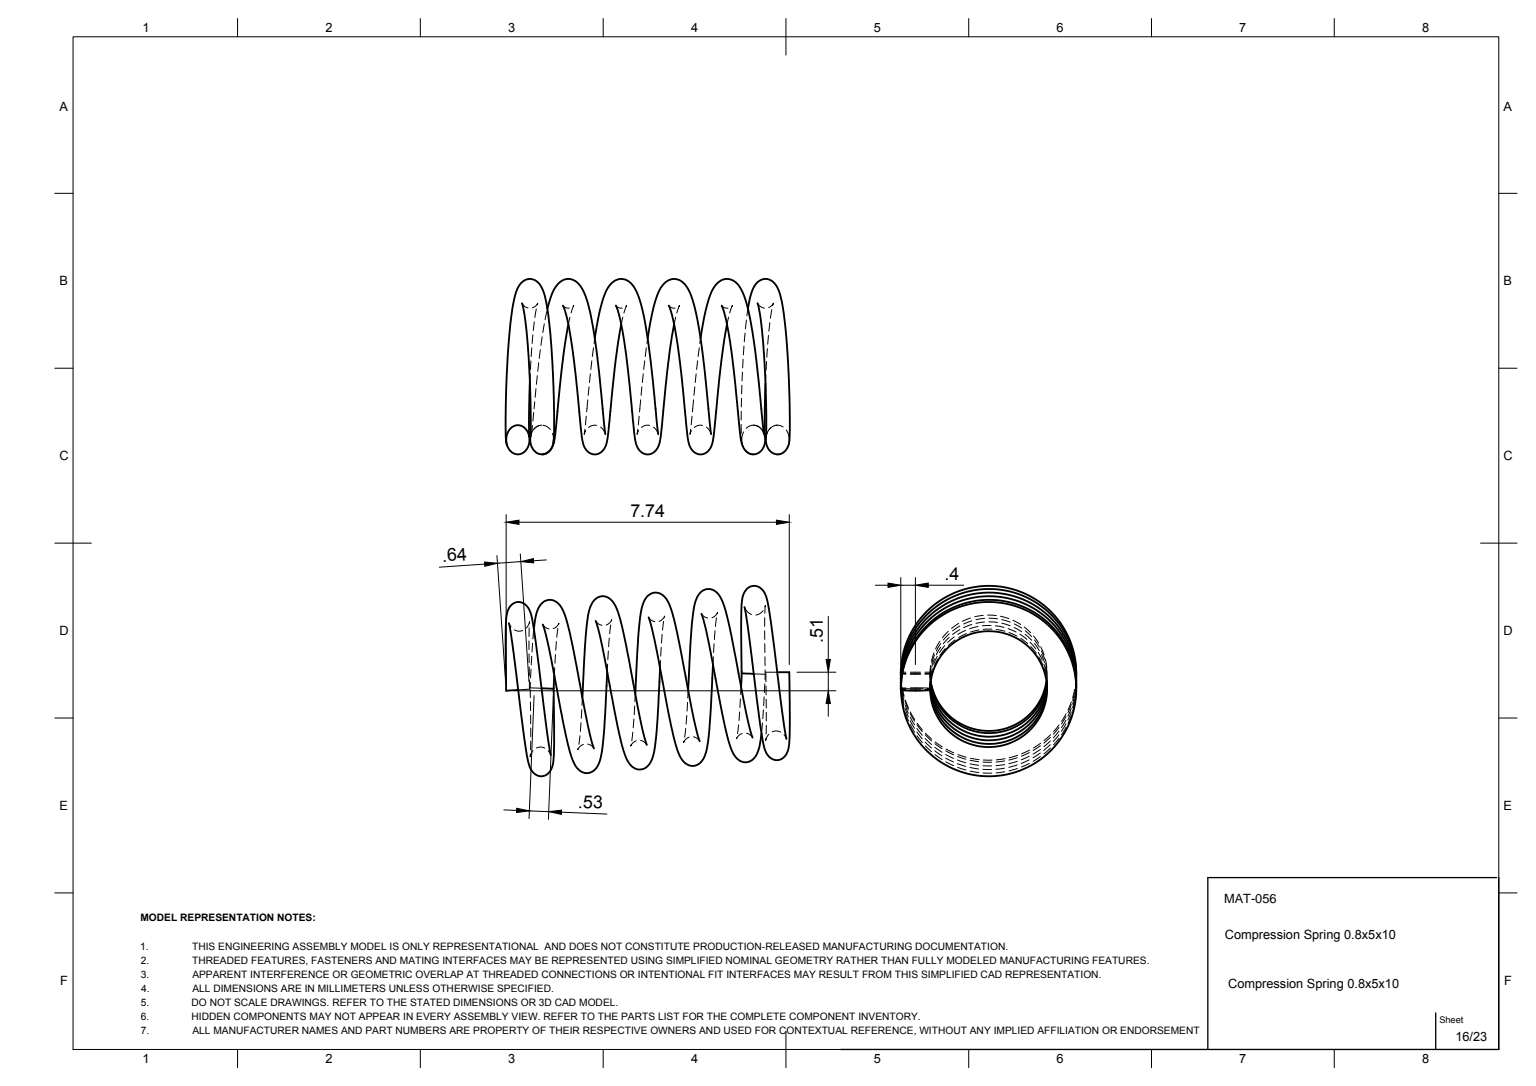
ISO-10303-21;
HEADER;
/* Generated by software containing ST-Developer
 * from STEP Tools, Inc. (www.steptools.com) 
 */

FILE_DESCRIPTION(
/* description */ (''),
/* implementation_level */ '2;1');

FILE_NAME(
/* name */ 'Compression Spring 0.8x5x10.step',
/* time_stamp */ '2026-10-28T16:47:13+01:00',
/* author */ (''),
/* organization */ (''),
/* preprocessor_version */ 'ST-DEVELOPER v20.2',
/* originating_system */ 'Autodesk Translation Framework v15.17.0.0',
/* authorisation */ '');

FILE_SCHEMA (('AUTOMOTIVE_DESIGN { 1 0 10303 214 3 1 1 }'));
ENDSEC;

DATA;
#10=MECHANICAL_DESIGN_GEOMETRIC_PRESENTATION_REPRESENTATION('',(#4588),#459242);
#186=ELLIPSE('',#99155,0.40000000018352,0.321902553589955);
#187=ELLIPSE('',#99156,0.400000000332434,0.321319291807333);
#188=ELLIPSE('',#99157,0.40000000018352,0.321902553589955);
#189=ELLIPSE('',#99158,0.400000000010015,0.321902553729585);
#190=ELLIPSE('',#99159,0.400000000010015,0.321902553729585);
#191=ELLIPSE('',#99160,0.4,0.32);
#192=ELLIPSE('',#99161,0.4,0.32);
#193=ELLIPSE('',#99162,0.400000000010016,0.321902553729585);
#194=ELLIPSE('',#99163,0.400000000010016,0.321902553729585);
#195=ELLIPSE('',#99165,0.400000000183514,0.321902553589955);
#196=ELLIPSE('',#99166,0.400000000183514,0.321902553589955);
#197=ELLIPSE('',#99168,0.40000000033243,0.321319291807334);
#2309=(
BOUNDED_SURFACE()
B_SPLINE_SURFACE(3,3,((#363644,#363645,#363646,#363647,#363648,#363649,
#363650,#363651,#363652,#363653,#363654,#363655,#363656,#363657,#363658,
#363659,#363660,#363661,#363662,#363663,#363664,#363665,#363666,#363667,
#363668,#363669,#363670,#363671,#363672),(#363673,#363674,#363675,#363676,
#363677,#363678,#363679,#363680,#363681,#363682,#363683,#363684,#363685,
#363686,#363687,#363688,#363689,#363690,#363691,#363692,#363693,#363694,
#363695,#363696,#363697,#363698,#363699,#363700,#363701),(#363702,#363703,
#363704,#363705,#363706,#363707,#363708,#363709,#363710,#363711,#363712,
#363713,#363714,#363715,#363716,#363717,#363718,#363719,#363720,#363721,
#363722,#363723,#363724,#363725,#363726,#363727,#363728,#363729,#363730),
(#363731,#363732,#363733,#363734,#363735,#363736,#363737,#363738,#363739,
#363740,#363741,#363742,#363743,#363744,#363745,#363746,#363747,#363748,
#363749,#363750,#363751,#363752,#363753,#363754,#363755,#363756,#363757,
#363758,#363759),(#363760,#363761,#363762,#363763,#363764,#363765,#363766,
#363767,#363768,#363769,#363770,#363771,#363772,#363773,#363774,#363775,
#363776,#363777,#363778,#363779,#363780,#363781,#363782,#363783,#363784,
#363785,#363786,#363787,#363788),(#363789,#363790,#363791,#363792,#363793,
#363794,#363795,#363796,#363797,#363798,#363799,#363800,#363801,#363802,
#363803,#363804,#363805,#363806,#363807,#363808,#363809,#363810,#363811,
#363812,#363813,#363814,#363815,#363816,#363817),(#363818,#363819,#363820,
#363821,#363822,#363823,#363824,#363825,#363826,#363827,#363828,#363829,
#363830,#363831,#363832,#363833,#363834,#363835,#363836,#363837,#363838,
#363839,#363840,#363841,#363842,#363843,#363844,#363845,#363846)),
 .UNSPECIFIED.,.T.,.F.,.F.)
B_SPLINE_SURFACE_WITH_KNOTS((4,3,4),(4,1,1,1,1,1,1,1,1,1,1,1,1,1,1,1,1,
1,1,1,1,1,1,1,1,1,4),(0.,0.5,1.),(0.,0.0310703336761616,0.0624385278003938,
0.0937144048499659,0.124978469089869,0.166663774179581,0.208294236860357,
0.249966520356582,0.291641529650434,0.3332733240007,0.374947073344913,0.416620808022619,
0.458253030541402,0.499926784452264,0.54160045129851,0.583232674441905,
0.624906496125386,0.666580158626562,0.708211959489969,0.749887054558503,
0.791559255246094,0.833189756589646,0.87487513422873,0.906139159779086,
0.937415106668169,0.968783217665703,1.),.UNSPECIFIED.)
GEOMETRIC_REPRESENTATION_ITEM()
RATIONAL_B_SPLINE_SURFACE(((1.,1.,1.,1.,1.,1.,1.,1.,1.,1.,1.,1.,1.,1.,1.,
1.,1.,1.,1.,1.,1.,1.,1.,1.,1.,1.,1.,1.,1.),(0.333333333333333,0.333333333333333,
0.333333333333334,0.333333333333333,0.333333333333333,0.333333333333333,
0.333333333333333,0.333333333333333,0.333333333333333,0.333333333333333,
0.333333333333333,0.333333333333333,0.333333333333334,0.333333333333333,
0.333333333333333,0.333333333333333,0.333333333333333,0.333333333333333,
0.333333333333333,0.333333333333333,0.333333333333333,0.333333333333333,
0.333333333333333,0.333333333333333,0.333333333333333,0.333333333333333,
0.333333333333333,0.333333333333333,0.333333333333333),(0.333333333333333,
0.333333333333333,0.333333333333334,0.333333333333333,0.333333333333333,
0.333333333333333,0.333333333333333,0.333333333333333,0.333333333333333,
0.333333333333333,0.333333333333333,0.333333333333333,0.333333333333334,
0.333333333333333,0.333333333333333,0.333333333333333,0.333333333333333,
0.333333333333333,0.333333333333333,0.333333333333333,0.333333333333333,
0.333333333333333,0.333333333333333,0.333333333333333,0.333333333333333,
0.333333333333333,0.333333333333333,0.333333333333333,0.333333333333333),
(1.,1.,1.,1.,1.,1.,1.,1.,1.,1.,1.,1.,1.,1.,1.,1.,1.,1.,1.,1.,1.,1.,1.,1.,
1.,1.,1.,1.,1.),(0.333333333333333,0.333333333333333,0.333333333333334,
0.333333333333333,0.333333333333333,0.333333333333333,0.333333333333333,
0.333333333333333,0.333333333333333,0.333333333333333,0.333333333333333,
0.333333333333333,0.333333333333334,0.333333333333333,0.333333333333333,
0.333333333333333,0.333333333333333,0.333333333333333,0.333333333333333,
0.333333333333333,0.333333333333333,0.333333333333333,0.333333333333333,
0.333333333333333,0.333333333333333,0.333333333333333,0.333333333333333,
0.333333333333333,0.333333333333333),(0.333333333333333,0.333333333333333,
0.333333333333334,0.333333333333333,0.333333333333333,0.333333333333333,
0.333333333333333,0.333333333333333,0.333333333333333,0.333333333333333,
0.333333333333333,0.333333333333333,0.333333333333334,0.333333333333333,
0.333333333333333,0.333333333333333,0.333333333333333,0.333333333333333,
0.333333333333333,0.333333333333333,0.333333333333333,0.333333333333333,
0.333333333333333,0.333333333333333,0.333333333333333,0.333333333333333,
0.333333333333333,0.333333333333333,0.333333333333333),(1.,1.,1.,1.,1.,
1.,1.,1.,1.,1.,1.,1.,1.,1.,1.,1.,1.,1.,1.,1.,1.,1.,1.,1.,1.,1.,1.,1.,1.)))
REPRESENTATION_ITEM('')
SURFACE()
);
#2310=(
BOUNDED_SURFACE()
B_SPLINE_SURFACE(3,3,((#363913,#363914,#363915,#363916,#363917,#363918,
#363919,#363920,#363921,#363922,#363923,#363924,#363925,#363926,#363927,
#363928,#363929,#363930,#363931,#363932,#363933,#363934,#363935,#363936,
#363937,#363938,#363939,#363940,#363941,#363942,#363943,#363944,#363945,
#363946,#363947,#363948,#363949,#363950,#363951,#363952,#363953,#363954,
#363955,#363956,#363957,#363958,#363959,#363960,#363961,#363962,#363963,
#363964,#363965,#363966,#363967,#363968,#363969,#363970,#363971,#363972,
#363973,#363974,#363975,#363976,#363977,#363978,#363979,#363980,#363981,
#363982,#363983,#363984,#363985,#363986,#363987,#363988,#363989,#363990,
#363991,#363992,#363993,#363994,#363995,#363996,#363997,#363998,#363999,
#364000,#364001,#364002,#364003,#364004,#364005,#364006,#364007,#364008,
#364009,#364010,#364011),(#364012,#364013,#364014,#364015,#364016,#364017,
#364018,#364019,#364020,#364021,#364022,#364023,#364024,#364025,#364026,
#364027,#364028,#364029,#364030,#364031,#364032,#364033,#364034,#364035,
#364036,#364037,#364038,#364039,#364040,#364041,#364042,#364043,#364044,
#364045,#364046,#364047,#364048,#364049,#364050,#364051,#364052,#364053,
#364054,#364055,#364056,#364057,#364058,#364059,#364060,#364061,#364062,
#364063,#364064,#364065,#364066,#364067,#364068,#364069,#364070,#364071,
#364072,#364073,#364074,#364075,#364076,#364077,#364078,#364079,#364080,
#364081,#364082,#364083,#364084,#364085,#364086,#364087,#364088,#364089,
#364090,#364091,#364092,#364093,#364094,#364095,#364096,#364097,#364098,
#364099,#364100,#364101,#364102,#364103,#364104,#364105,#364106,#364107,
#364108,#364109,#364110),(#364111,#364112,#364113,#364114,#364115,#364116,
#364117,#364118,#364119,#364120,#364121,#364122,#364123,#364124,#364125,
#364126,#364127,#364128,#364129,#364130,#364131,#364132,#364133,#364134,
#364135,#364136,#364137,#364138,#364139,#364140,#364141,#364142,#364143,
#364144,#364145,#364146,#364147,#364148,#364149,#364150,#364151,#364152,
#364153,#364154,#364155,#364156,#364157,#364158,#364159,#364160,#364161,
#364162,#364163,#364164,#364165,#364166,#364167,#364168,#364169,#364170,
#364171,#364172,#364173,#364174,#364175,#364176,#364177,#364178,#364179,
#364180,#364181,#364182,#364183,#364184,#364185,#364186,#364187,#364188,
#364189,#364190,#364191,#364192,#364193,#364194,#364195,#364196,#364197,
#364198,#364199,#364200,#364201,#364202,#364203,#364204,#364205,#364206,
#364207,#364208,#364209),(#364210,#364211,#364212,#364213,#364214,#364215,
#364216,#364217,#364218,#364219,#364220,#364221,#364222,#364223,#364224,
#364225,#364226,#364227,#364228,#364229,#364230,#364231,#364232,#364233,
#364234,#364235,#364236,#364237,#364238,#364239,#364240,#364241,#364242,
#364243,#364244,#364245,#364246,#364247,#364248,#364249,#364250,#364251,
#364252,#364253,#364254,#364255,#364256,#364257,#364258,#364259,#364260,
#364261,#364262,#364263,#364264,#364265,#364266,#364267,#364268,#364269,
#364270,#364271,#364272,#364273,#364274,#364275,#364276,#364277,#364278,
#364279,#364280,#364281,#364282,#364283,#364284,#364285,#364286,#364287,
#364288,#364289,#364290,#364291,#364292,#364293,#364294,#364295,#364296,
#364297,#364298,#364299,#364300,#364301,#364302,#364303,#364304,#364305,
#364306,#364307,#364308),(#364309,#364310,#364311,#364312,#364313,#364314,
#364315,#364316,#364317,#364318,#364319,#364320,#364321,#364322,#364323,
#364324,#364325,#364326,#364327,#364328,#364329,#364330,#364331,#364332,
#364333,#364334,#364335,#364336,#364337,#364338,#364339,#364340,#364341,
#364342,#364343,#364344,#364345,#364346,#364347,#364348,#364349,#364350,
#364351,#364352,#364353,#364354,#364355,#364356,#364357,#364358,#364359,
#364360,#364361,#364362,#364363,#364364,#364365,#364366,#364367,#364368,
#364369,#364370,#364371,#364372,#364373,#364374,#364375,#364376,#364377,
#364378,#364379,#364380,#364381,#364382,#364383,#364384,#364385,#364386,
#364387,#364388,#364389,#364390,#364391,#364392,#364393,#364394,#364395,
#364396,#364397,#364398,#364399,#364400,#364401,#364402,#364403,#364404,
#364405,#364406,#364407),(#364408,#364409,#364410,#364411,#364412,#364413,
#364414,#364415,#364416,#364417,#364418,#364419,#364420,#364421,#364422,
#364423,#364424,#364425,#364426,#364427,#364428,#364429,#364430,#364431,
#364432,#364433,#364434,#364435,#364436,#364437,#364438,#364439,#364440,
#364441,#364442,#364443,#364444,#364445,#364446,#364447,#364448,#364449,
#364450,#364451,#364452,#364453,#364454,#364455,#364456,#364457,#364458,
#364459,#364460,#364461,#364462,#364463,#364464,#364465,#364466,#364467,
#364468,#364469,#364470,#364471,#364472,#364473,#364474,#364475,#364476,
#364477,#364478,#364479,#364480,#364481,#364482,#364483,#364484,#364485,
#364486,#364487,#364488,#364489,#364490,#364491,#364492,#364493,#364494,
#364495,#364496,#364497,#364498,#364499,#364500,#364501,#364502,#364503,
#364504,#364505,#364506),(#364507,#364508,#364509,#364510,#364511,#364512,
#364513,#364514,#364515,#364516,#364517,#364518,#364519,#364520,#364521,
#364522,#364523,#364524,#364525,#364526,#364527,#364528,#364529,#364530,
#364531,#364532,#364533,#364534,#364535,#364536,#364537,#364538,#364539,
#364540,#364541,#364542,#364543,#364544,#364545,#364546,#364547,#364548,
#364549,#364550,#364551,#364552,#364553,#364554,#364555,#364556,#364557,
#364558,#364559,#364560,#364561,#364562,#364563,#364564,#364565,#364566,
#364567,#364568,#364569,#364570,#364571,#364572,#364573,#364574,#364575,
#364576,#364577,#364578,#364579,#364580,#364581,#364582,#364583,#364584,
#364585,#364586,#364587,#364588,#364589,#364590,#364591,#364592,#364593,
#364594,#364595,#364596,#364597,#364598,#364599,#364600,#364601,#364602,
#364603,#364604,#364605)),.UNSPECIFIED.,.T.,.F.,.F.)
B_SPLINE_SURFACE_WITH_KNOTS((4,3,4),(4,1,1,1,1,1,1,1,1,1,1,1,1,1,1,1,1,
1,1,1,1,1,1,1,1,1,1,1,1,1,1,1,1,1,1,1,1,1,1,1,1,1,1,1,1,1,1,1,1,1,1,1,1,
1,1,1,1,1,1,1,1,1,1,1,1,1,1,1,1,1,1,1,1,1,1,1,1,1,1,1,1,1,1,1,1,1,1,1,1,
1,1,1,1,1,1,1,4),(0.,0.5,1.),(0.,0.0104467457848562,0.0208697051534179,
0.0312830741812588,0.0417059245369557,0.0521151844214314,0.0625350854994869,
0.072955523619078,0.0833651614361216,0.093785355257659,0.104205506224069,
0.114615259182489,0.125035444608255,0.135455580151817,0.145865343296126,
0.156285526040368,0.166705661591602,0.177115425208493,0.187535607700786,
0.197955743339009,0.208365506953668,0.218785689432554,0.229205825080053,
0.239615588692213,0.250035771170918,0.260455906818944,0.270865670430874,
0.281285852909622,0.291705988557657,0.302115752169577,0.312535934648329,
0.322956070296362,0.333365833908282,0.343786016387035,0.354206152035067,
0.364615915646988,0.375036098125741,0.385456233773773,0.395865997385694,
0.406286179864446,0.416706315512479,0.427116079124399,0.437536261603152,
0.447956397251184,0.458366160863105,0.468786343341857,0.47920647898989,
0.48961624260181,0.500036425080563,0.510456560728595,0.520866324340516,
0.531286506819269,0.541706642467301,0.552116406079222,0.562536588557974,
0.572956724206007,0.583366487817927,0.59378667029668,0.604206805944712,
0.614616569556633,0.625036752035385,0.635456887683418,0.645866651295338,
0.656286833774091,0.666706969422123,0.677116733034044,0.687536915512797,
0.697957051160829,0.708366814772749,0.718786997251504,0.729207132899531,
0.739616896511461,0.750037078990207,0.760457214638192,0.770866978250353,
0.781287160728572,0.791707296376735,0.802117059991444,0.812537242460403,
0.822957378121908,0.833367141740239,0.843787324122365,0.85420746003523,
0.864617223206175,0.875037405580635,0.885457544175532,0.895867297492078,
0.906287495257385,0.916707642366043,0.927117283641006,0.937537767903979,
0.947957624414904,0.958366904818021,0.968789794286159,0.979203137018726,
0.989626134310512,1.),.UNSPECIFIED.)
GEOMETRIC_REPRESENTATION_ITEM()
RATIONAL_B_SPLINE_SURFACE(((1.,1.,1.,1.,1.,1.,1.,1.,1.,1.,1.,1.,1.,1.,1.,
1.,1.,1.,1.,1.,1.,1.,1.,1.,1.,1.,1.,1.,1.,1.,1.,1.,1.,1.,1.,1.,1.,1.,1.,
1.,1.,1.,1.,1.,1.,1.,1.,1.,1.,1.,1.,1.,1.,1.,1.,1.,1.,1.,1.,1.,1.,1.,1.,
1.,1.,1.,1.,1.,1.,1.,1.,1.,1.,1.,1.,1.,1.,1.,1.,1.,1.,1.,1.,1.,1.,1.,1.,
1.,1.,1.,1.,1.,1.,1.,1.,1.,1.,1.,1.),(0.333333333333333,0.333333333333333,
0.333333333333333,0.333333333333333,0.333333333333333,0.333333333333333,
0.333333333333333,0.333333333333333,0.333333333333333,0.333333333333333,
0.333333333333333,0.333333333333333,0.333333333333333,0.333333333333333,
0.333333333333333,0.333333333333333,0.333333333333333,0.333333333333333,
0.333333333333333,0.333333333333333,0.333333333333333,0.333333333333333,
0.333333333333333,0.333333333333333,0.333333333333333,0.333333333333333,
0.333333333333333,0.333333333333333,0.333333333333333,0.333333333333333,
0.333333333333333,0.333333333333333,0.333333333333333,0.333333333333333,
0.333333333333333,0.333333333333333,0.333333333333333,0.333333333333333,
0.333333333333333,0.333333333333333,0.333333333333333,0.333333333333333,
0.333333333333333,0.333333333333333,0.333333333333333,0.333333333333333,
0.333333333333333,0.333333333333333,0.333333333333333,0.333333333333333,
0.333333333333333,0.333333333333333,0.333333333333333,0.333333333333333,
0.333333333333333,0.333333333333333,0.333333333333333,0.333333333333333,
0.333333333333333,0.333333333333333,0.333333333333333,0.333333333333333,
0.333333333333333,0.333333333333333,0.333333333333333,0.333333333333333,
0.333333333333333,0.333333333333333,0.333333333333333,0.333333333333333,
0.333333333333333,0.333333333333333,0.333333333333333,0.333333333333333,
0.333333333333333,0.333333333333333,0.333333333333333,0.333333333333333,
0.333333333333333,0.333333333333333,0.333333333333333,0.333333333333333,
0.333333333333333,0.333333333333333,0.333333333333333,0.333333333333333,
0.333333333333333,0.333333333333333,0.333333333333333,0.333333333333333,
0.333333333333333,0.333333333333333,0.333333333333333,0.333333333333333,
0.333333333333333,0.333333333333333,0.333333333333333,0.333333333333333,
0.333333333333333),(0.333333333333333,0.333333333333333,0.333333333333333,
0.333333333333333,0.333333333333333,0.333333333333333,0.333333333333333,
0.333333333333333,0.333333333333333,0.333333333333333,0.333333333333333,
0.333333333333333,0.333333333333333,0.333333333333333,0.333333333333333,
0.333333333333333,0.333333333333333,0.333333333333333,0.333333333333333,
0.333333333333333,0.333333333333333,0.333333333333333,0.333333333333333,
0.333333333333333,0.333333333333333,0.333333333333333,0.333333333333333,
0.333333333333333,0.333333333333333,0.333333333333333,0.333333333333333,
0.333333333333333,0.333333333333333,0.333333333333333,0.333333333333333,
0.333333333333333,0.333333333333333,0.333333333333333,0.333333333333333,
0.333333333333333,0.333333333333333,0.333333333333333,0.333333333333333,
0.333333333333333,0.333333333333333,0.333333333333333,0.333333333333333,
0.333333333333333,0.333333333333333,0.333333333333333,0.333333333333333,
0.333333333333333,0.333333333333333,0.333333333333333,0.333333333333333,
0.333333333333333,0.333333333333333,0.333333333333333,0.333333333333333,
0.333333333333333,0.333333333333333,0.333333333333333,0.333333333333333,
0.333333333333333,0.333333333333333,0.333333333333333,0.333333333333333,
0.333333333333333,0.333333333333333,0.333333333333333,0.333333333333333,
0.333333333333333,0.333333333333333,0.333333333333333,0.333333333333333,
0.333333333333333,0.333333333333333,0.333333333333333,0.333333333333333,
0.333333333333333,0.333333333333333,0.333333333333333,0.333333333333333,
0.333333333333333,0.333333333333333,0.333333333333333,0.333333333333333,
0.333333333333333,0.333333333333333,0.333333333333333,0.333333333333333,
0.333333333333333,0.333333333333333,0.333333333333333,0.333333333333333,
0.333333333333333,0.333333333333333,0.333333333333333,0.333333333333333),
(1.,1.,1.,1.,1.,1.,1.,1.,1.,1.,1.,1.,1.,1.,1.,1.,1.,1.,1.,1.,1.,1.,1.,1.,
1.,1.,1.,1.,1.,1.,1.,1.,1.,1.,1.,1.,1.,1.,1.,1.,1.,1.,1.,1.,1.,1.,1.,1.,
1.,1.,1.,1.,1.,1.,1.,1.,1.,1.,1.,1.,1.,1.,1.,1.,1.,1.,1.,1.,1.,1.,1.,1.,
1.,1.,1.,1.,1.,1.,1.,1.,1.,1.,1.,1.,1.,1.,1.,1.,1.,1.,1.,1.,1.,1.,1.,1.,
1.,1.,1.),(0.333333333333333,0.333333333333333,0.333333333333333,0.333333333333333,
0.333333333333333,0.333333333333333,0.333333333333333,0.333333333333333,
0.333333333333333,0.333333333333333,0.333333333333333,0.333333333333333,
0.333333333333333,0.333333333333333,0.333333333333333,0.333333333333333,
0.333333333333333,0.333333333333333,0.333333333333333,0.333333333333333,
0.333333333333333,0.333333333333333,0.333333333333333,0.333333333333333,
0.333333333333333,0.333333333333333,0.333333333333333,0.333333333333333,
0.333333333333333,0.333333333333333,0.333333333333333,0.333333333333333,
0.333333333333333,0.333333333333333,0.333333333333333,0.333333333333333,
0.333333333333333,0.333333333333333,0.333333333333333,0.333333333333333,
0.333333333333333,0.333333333333333,0.333333333333333,0.333333333333333,
0.333333333333333,0.333333333333333,0.333333333333333,0.333333333333333,
0.333333333333333,0.333333333333333,0.333333333333333,0.333333333333333,
0.333333333333333,0.333333333333333,0.333333333333333,0.333333333333333,
0.333333333333333,0.333333333333333,0.333333333333333,0.333333333333333,
0.333333333333333,0.333333333333333,0.333333333333333,0.333333333333333,
0.333333333333333,0.333333333333333,0.333333333333333,0.333333333333333,
0.333333333333333,0.333333333333333,0.333333333333333,0.333333333333333,
0.333333333333333,0.333333333333333,0.333333333333333,0.333333333333333,
0.333333333333333,0.333333333333333,0.333333333333333,0.333333333333333,
0.333333333333333,0.333333333333333,0.333333333333333,0.333333333333333,
0.333333333333333,0.333333333333333,0.333333333333333,0.333333333333333,
0.333333333333333,0.333333333333333,0.333333333333333,0.333333333333333,
0.333333333333333,0.333333333333333,0.333333333333333,0.333333333333333,
0.333333333333333,0.333333333333333,0.333333333333333),(0.333333333333333,
0.333333333333333,0.333333333333333,0.333333333333333,0.333333333333333,
0.333333333333333,0.333333333333333,0.333333333333333,0.333333333333333,
0.333333333333333,0.333333333333333,0.333333333333333,0.333333333333333,
0.333333333333333,0.333333333333333,0.333333333333333,0.333333333333333,
0.333333333333333,0.333333333333333,0.333333333333333,0.333333333333333,
0.333333333333333,0.333333333333333,0.333333333333333,0.333333333333333,
0.333333333333333,0.333333333333333,0.333333333333333,0.333333333333333,
0.333333333333333,0.333333333333333,0.333333333333333,0.333333333333333,
0.333333333333333,0.333333333333333,0.333333333333333,0.333333333333333,
0.333333333333333,0.333333333333333,0.333333333333333,0.333333333333333,
0.333333333333333,0.333333333333333,0.333333333333333,0.333333333333333,
0.333333333333333,0.333333333333333,0.333333333333333,0.333333333333333,
0.333333333333333,0.333333333333333,0.333333333333333,0.333333333333333,
0.333333333333333,0.333333333333333,0.333333333333333,0.333333333333333,
0.333333333333333,0.333333333333333,0.333333333333333,0.333333333333333,
0.333333333333333,0.333333333333333,0.333333333333333,0.333333333333333,
0.333333333333333,0.333333333333333,0.333333333333333,0.333333333333333,
0.333333333333333,0.333333333333333,0.333333333333333,0.333333333333333,
0.333333333333333,0.333333333333333,0.333333333333333,0.333333333333333,
0.333333333333333,0.333333333333333,0.333333333333333,0.333333333333333,
0.333333333333333,0.333333333333333,0.333333333333333,0.333333333333333,
0.333333333333333,0.333333333333333,0.333333333333333,0.333333333333333,
0.333333333333333,0.333333333333333,0.333333333333333,0.333333333333333,
0.333333333333333,0.333333333333333,0.333333333333333,0.333333333333333,
0.333333333333333,0.333333333333333),(1.,1.,1.,1.,1.,1.,1.,1.,1.,1.,1.,
1.,1.,1.,1.,1.,1.,1.,1.,1.,1.,1.,1.,1.,1.,1.,1.,1.,1.,1.,1.,1.,1.,1.,1.,
1.,1.,1.,1.,1.,1.,1.,1.,1.,1.,1.,1.,1.,1.,1.,1.,1.,1.,1.,1.,1.,1.,1.,1.,
1.,1.,1.,1.,1.,1.,1.,1.,1.,1.,1.,1.,1.,1.,1.,1.,1.,1.,1.,1.,1.,1.,1.,1.,
1.,1.,1.,1.,1.,1.,1.,1.,1.,1.,1.,1.,1.,1.,1.,1.)))
REPRESENTATION_ITEM('')
SURFACE()
);
#2311=(
BOUNDED_SURFACE()
B_SPLINE_SURFACE(3,3,((#364809,#364810,#364811,#364812,#364813,#364814,
#364815,#364816,#364817,#364818,#364819,#364820,#364821,#364822,#364823,
#364824,#364825,#364826,#364827,#364828,#364829,#364830,#364831,#364832,
#364833,#364834,#364835,#364836,#364837),(#364838,#364839,#364840,#364841,
#364842,#364843,#364844,#364845,#364846,#364847,#364848,#364849,#364850,
#364851,#364852,#364853,#364854,#364855,#364856,#364857,#364858,#364859,
#364860,#364861,#364862,#364863,#364864,#364865,#364866),(#364867,#364868,
#364869,#364870,#364871,#364872,#364873,#364874,#364875,#364876,#364877,
#364878,#364879,#364880,#364881,#364882,#364883,#364884,#364885,#364886,
#364887,#364888,#364889,#364890,#364891,#364892,#364893,#364894,#364895),
(#364896,#364897,#364898,#364899,#364900,#364901,#364902,#364903,#364904,
#364905,#364906,#364907,#364908,#364909,#364910,#364911,#364912,#364913,
#364914,#364915,#364916,#364917,#364918,#364919,#364920,#364921,#364922,
#364923,#364924),(#364925,#364926,#364927,#364928,#364929,#364930,#364931,
#364932,#364933,#364934,#364935,#364936,#364937,#364938,#364939,#364940,
#364941,#364942,#364943,#364944,#364945,#364946,#364947,#364948,#364949,
#364950,#364951,#364952,#364953),(#364954,#364955,#364956,#364957,#364958,
#364959,#364960,#364961,#364962,#364963,#364964,#364965,#364966,#364967,
#364968,#364969,#364970,#364971,#364972,#364973,#364974,#364975,#364976,
#364977,#364978,#364979,#364980,#364981,#364982),(#364983,#364984,#364985,
#364986,#364987,#364988,#364989,#364990,#364991,#364992,#364993,#364994,
#364995,#364996,#364997,#364998,#364999,#365000,#365001,#365002,#365003,
#365004,#365005,#365006,#365007,#365008,#365009,#365010,#365011)),
 .UNSPECIFIED.,.T.,.F.,.F.)
B_SPLINE_SURFACE_WITH_KNOTS((4,3,4),(4,1,1,1,1,1,1,1,1,1,1,1,1,1,1,1,1,
1,1,1,1,1,1,1,1,1,4),(0.,0.5,1.),(0.,0.0311997468912562,0.0625509890871527,
0.0938098447846757,0.1250568872711,0.166719530856106,0.208327420639085,
0.249977065870109,0.291629399375196,0.333238604634684,0.374889730322128,
0.41654078485731,0.458150415717,0.499801548056339,0.541452534012182,0.583062165488229,
0.624713366295055,0.666364346005318,0.707973557473876,0.749626035232519,
0.791275541260273,0.832883464833855,0.874546235186119,0.905793212129613,
0.937052173453026,0.968403278656631,1.),.UNSPECIFIED.)
GEOMETRIC_REPRESENTATION_ITEM()
RATIONAL_B_SPLINE_SURFACE(((1.,1.,1.,1.,1.,1.,1.,1.,1.,1.,1.,1.,1.,1.,1.,
1.,1.,1.,1.,1.,1.,1.,1.,1.,1.,1.,1.,1.,1.),(0.333333333333333,0.333333333333333,
0.333333333333333,0.333333333333333,0.333333333333333,0.333333333333333,
0.333333333333334,0.333333333333333,0.333333333333333,0.333333333333333,
0.333333333333333,0.333333333333333,0.333333333333333,0.333333333333334,
0.333333333333333,0.333333333333333,0.333333333333333,0.333333333333333,
0.333333333333333,0.333333333333333,0.333333333333333,0.333333333333333,
0.333333333333333,0.333333333333333,0.333333333333334,0.333333333333333,
0.333333333333333,0.333333333333333,0.333333333333333),(0.333333333333333,
0.333333333333333,0.333333333333333,0.333333333333333,0.333333333333333,
0.333333333333333,0.333333333333334,0.333333333333333,0.333333333333333,
0.333333333333333,0.333333333333333,0.333333333333333,0.333333333333333,
0.333333333333334,0.333333333333333,0.333333333333333,0.333333333333333,
0.333333333333333,0.333333333333333,0.333333333333333,0.333333333333333,
0.333333333333333,0.333333333333333,0.333333333333333,0.333333333333334,
0.333333333333333,0.333333333333333,0.333333333333333,0.333333333333333),
(1.,1.,1.,1.,1.,1.,1.,1.,1.,1.,1.,1.,1.,1.,1.,1.,1.,1.,1.,1.,1.,1.,1.,1.,
1.,1.,1.,1.,1.),(0.333333333333333,0.333333333333333,0.333333333333333,
0.333333333333333,0.333333333333333,0.333333333333333,0.333333333333334,
0.333333333333333,0.333333333333333,0.333333333333333,0.333333333333333,
0.333333333333333,0.333333333333333,0.333333333333334,0.333333333333333,
0.333333333333333,0.333333333333333,0.333333333333333,0.333333333333333,
0.333333333333333,0.333333333333333,0.333333333333333,0.333333333333333,
0.333333333333333,0.333333333333334,0.333333333333333,0.333333333333333,
0.333333333333333,0.333333333333333),(0.333333333333333,0.333333333333333,
0.333333333333333,0.333333333333333,0.333333333333333,0.333333333333333,
0.333333333333334,0.333333333333333,0.333333333333333,0.333333333333333,
0.333333333333333,0.333333333333333,0.333333333333333,0.333333333333334,
0.333333333333333,0.333333333333333,0.333333333333333,0.333333333333333,
0.333333333333333,0.333333333333333,0.333333333333333,0.333333333333333,
0.333333333333333,0.333333333333333,0.333333333333334,0.333333333333333,
0.333333333333333,0.333333333333333,0.333333333333333),(1.,1.,1.,1.,1.,
1.,1.,1.,1.,1.,1.,1.,1.,1.,1.,1.,1.,1.,1.,1.,1.,1.,1.,1.,1.,1.,1.,1.,1.)))
REPRESENTATION_ITEM('')
SURFACE()
);
#2312=(
BOUNDED_SURFACE()
B_SPLINE_SURFACE(3,3,((#365073,#365074,#365075,#365076,#365077,#365078,
#365079,#365080,#365081,#365082,#365083,#365084,#365085,#365086,#365087,
#365088,#365089,#365090,#365091,#365092,#365093,#365094,#365095,#365096,
#365097,#365098,#365099,#365100,#365101),(#365102,#365103,#365104,#365105,
#365106,#365107,#365108,#365109,#365110,#365111,#365112,#365113,#365114,
#365115,#365116,#365117,#365118,#365119,#365120,#365121,#365122,#365123,
#365124,#365125,#365126,#365127,#365128,#365129,#365130),(#365131,#365132,
#365133,#365134,#365135,#365136,#365137,#365138,#365139,#365140,#365141,
#365142,#365143,#365144,#365145,#365146,#365147,#365148,#365149,#365150,
#365151,#365152,#365153,#365154,#365155,#365156,#365157,#365158,#365159),
(#365160,#365161,#365162,#365163,#365164,#365165,#365166,#365167,#365168,
#365169,#365170,#365171,#365172,#365173,#365174,#365175,#365176,#365177,
#365178,#365179,#365180,#365181,#365182,#365183,#365184,#365185,#365186,
#365187,#365188),(#365189,#365190,#365191,#365192,#365193,#365194,#365195,
#365196,#365197,#365198,#365199,#365200,#365201,#365202,#365203,#365204,
#365205,#365206,#365207,#365208,#365209,#365210,#365211,#365212,#365213,
#365214,#365215,#365216,#365217),(#365218,#365219,#365220,#365221,#365222,
#365223,#365224,#365225,#365226,#365227,#365228,#365229,#365230,#365231,
#365232,#365233,#365234,#365235,#365236,#365237,#365238,#365239,#365240,
#365241,#365242,#365243,#365244,#365245,#365246),(#365247,#365248,#365249,
#365250,#365251,#365252,#365253,#365254,#365255,#365256,#365257,#365258,
#365259,#365260,#365261,#365262,#365263,#365264,#365265,#365266,#365267,
#365268,#365269,#365270,#365271,#365272,#365273,#365274,#365275)),
 .UNSPECIFIED.,.T.,.F.,.F.)
B_SPLINE_SURFACE_WITH_KNOTS((4,3,4),(4,1,1,1,1,1,1,1,1,1,1,1,1,1,1,1,1,
1,1,1,1,1,1,1,1,1,4),(0.,0.5,1.),(0.,0.0311997468912562,0.0625509890871527,
0.0938098447846757,0.1250568872711,0.166719530856106,0.208327420639085,
0.249977065870109,0.291629399375196,0.333238604634684,0.374889730322128,
0.41654078485731,0.458150415717,0.499801548056339,0.541452534012182,0.583062165488229,
0.624713366295055,0.666364346005318,0.707973557473876,0.749626035232519,
0.791275541260273,0.832883464833855,0.874546235186119,0.905793212129613,
0.937052173453026,0.968403278656631,1.),.UNSPECIFIED.)
GEOMETRIC_REPRESENTATION_ITEM()
RATIONAL_B_SPLINE_SURFACE(((1.,1.,1.,1.,1.,1.,1.,1.,1.,1.,1.,1.,1.,1.,1.,
1.,1.,1.,1.,1.,1.,1.,1.,1.,1.,1.,1.,1.,1.),(0.333333333333333,0.333333333333333,
0.333333333333333,0.333333333333333,0.333333333333333,0.333333333333333,
0.333333333333334,0.333333333333333,0.333333333333333,0.333333333333333,
0.333333333333333,0.333333333333333,0.333333333333333,0.333333333333334,
0.333333333333333,0.333333333333333,0.333333333333333,0.333333333333333,
0.333333333333333,0.333333333333333,0.333333333333333,0.333333333333333,
0.333333333333333,0.333333333333333,0.333333333333334,0.333333333333333,
0.333333333333333,0.333333333333333,0.333333333333333),(0.333333333333333,
0.333333333333333,0.333333333333333,0.333333333333333,0.333333333333333,
0.333333333333333,0.333333333333334,0.333333333333333,0.333333333333333,
0.333333333333333,0.333333333333333,0.333333333333333,0.333333333333333,
0.333333333333334,0.333333333333333,0.333333333333333,0.333333333333333,
0.333333333333333,0.333333333333333,0.333333333333333,0.333333333333333,
0.333333333333333,0.333333333333333,0.333333333333333,0.333333333333334,
0.333333333333333,0.333333333333333,0.333333333333333,0.333333333333333),
(1.,1.,1.,1.,1.,1.,1.,1.,1.,1.,1.,1.,1.,1.,1.,1.,1.,1.,1.,1.,1.,1.,1.,1.,
1.,1.,1.,1.,1.),(0.333333333333333,0.333333333333333,0.333333333333333,
0.333333333333333,0.333333333333333,0.333333333333333,0.333333333333334,
0.333333333333333,0.333333333333333,0.333333333333333,0.333333333333333,
0.333333333333333,0.333333333333333,0.333333333333334,0.333333333333333,
0.333333333333333,0.333333333333333,0.333333333333333,0.333333333333333,
0.333333333333333,0.333333333333333,0.333333333333333,0.333333333333333,
0.333333333333333,0.333333333333334,0.333333333333333,0.333333333333333,
0.333333333333333,0.333333333333333),(0.333333333333333,0.333333333333333,
0.333333333333333,0.333333333333333,0.333333333333333,0.333333333333333,
0.333333333333334,0.333333333333333,0.333333333333333,0.333333333333333,
0.333333333333333,0.333333333333333,0.333333333333333,0.333333333333334,
0.333333333333333,0.333333333333333,0.333333333333333,0.333333333333333,
0.333333333333333,0.333333333333333,0.333333333333333,0.333333333333333,
0.333333333333333,0.333333333333333,0.333333333333334,0.333333333333333,
0.333333333333333,0.333333333333333,0.333333333333333),(1.,1.,1.,1.,1.,
1.,1.,1.,1.,1.,1.,1.,1.,1.,1.,1.,1.,1.,1.,1.,1.,1.,1.,1.,1.,1.,1.,1.,1.)))
REPRESENTATION_ITEM('')
SURFACE()
);
#2313=(
BOUNDED_SURFACE()
B_SPLINE_SURFACE(3,3,((#365281,#365282,#365283,#365284,#365285,#365286,
#365287,#365288,#365289,#365290,#365291,#365292,#365293,#365294,#365295,
#365296,#365297,#365298,#365299,#365300,#365301,#365302,#365303,#365304,
#365305,#365306,#365307,#365308,#365309,#365310,#365311,#365312,#365313,
#365314,#365315,#365316,#365317,#365318,#365319,#365320,#365321,#365322,
#365323,#365324,#365325,#365326,#365327,#365328,#365329,#365330,#365331,
#365332,#365333,#365334,#365335,#365336,#365337,#365338,#365339,#365340,
#365341,#365342,#365343,#365344,#365345,#365346,#365347,#365348,#365349,
#365350,#365351,#365352,#365353,#365354,#365355,#365356,#365357,#365358,
#365359,#365360,#365361,#365362,#365363,#365364,#365365,#365366,#365367,
#365368,#365369,#365370,#365371,#365372,#365373,#365374,#365375,#365376,
#365377,#365378,#365379),(#365380,#365381,#365382,#365383,#365384,#365385,
#365386,#365387,#365388,#365389,#365390,#365391,#365392,#365393,#365394,
#365395,#365396,#365397,#365398,#365399,#365400,#365401,#365402,#365403,
#365404,#365405,#365406,#365407,#365408,#365409,#365410,#365411,#365412,
#365413,#365414,#365415,#365416,#365417,#365418,#365419,#365420,#365421,
#365422,#365423,#365424,#365425,#365426,#365427,#365428,#365429,#365430,
#365431,#365432,#365433,#365434,#365435,#365436,#365437,#365438,#365439,
#365440,#365441,#365442,#365443,#365444,#365445,#365446,#365447,#365448,
#365449,#365450,#365451,#365452,#365453,#365454,#365455,#365456,#365457,
#365458,#365459,#365460,#365461,#365462,#365463,#365464,#365465,#365466,
#365467,#365468,#365469,#365470,#365471,#365472,#365473,#365474,#365475,
#365476,#365477,#365478),(#365479,#365480,#365481,#365482,#365483,#365484,
#365485,#365486,#365487,#365488,#365489,#365490,#365491,#365492,#365493,
#365494,#365495,#365496,#365497,#365498,#365499,#365500,#365501,#365502,
#365503,#365504,#365505,#365506,#365507,#365508,#365509,#365510,#365511,
#365512,#365513,#365514,#365515,#365516,#365517,#365518,#365519,#365520,
#365521,#365522,#365523,#365524,#365525,#365526,#365527,#365528,#365529,
#365530,#365531,#365532,#365533,#365534,#365535,#365536,#365537,#365538,
#365539,#365540,#365541,#365542,#365543,#365544,#365545,#365546,#365547,
#365548,#365549,#365550,#365551,#365552,#365553,#365554,#365555,#365556,
#365557,#365558,#365559,#365560,#365561,#365562,#365563,#365564,#365565,
#365566,#365567,#365568,#365569,#365570,#365571,#365572,#365573,#365574,
#365575,#365576,#365577),(#365578,#365579,#365580,#365581,#365582,#365583,
#365584,#365585,#365586,#365587,#365588,#365589,#365590,#365591,#365592,
#365593,#365594,#365595,#365596,#365597,#365598,#365599,#365600,#365601,
#365602,#365603,#365604,#365605,#365606,#365607,#365608,#365609,#365610,
#365611,#365612,#365613,#365614,#365615,#365616,#365617,#365618,#365619,
#365620,#365621,#365622,#365623,#365624,#365625,#365626,#365627,#365628,
#365629,#365630,#365631,#365632,#365633,#365634,#365635,#365636,#365637,
#365638,#365639,#365640,#365641,#365642,#365643,#365644,#365645,#365646,
#365647,#365648,#365649,#365650,#365651,#365652,#365653,#365654,#365655,
#365656,#365657,#365658,#365659,#365660,#365661,#365662,#365663,#365664,
#365665,#365666,#365667,#365668,#365669,#365670,#365671,#365672,#365673,
#365674,#365675,#365676),(#365677,#365678,#365679,#365680,#365681,#365682,
#365683,#365684,#365685,#365686,#365687,#365688,#365689,#365690,#365691,
#365692,#365693,#365694,#365695,#365696,#365697,#365698,#365699,#365700,
#365701,#365702,#365703,#365704,#365705,#365706,#365707,#365708,#365709,
#365710,#365711,#365712,#365713,#365714,#365715,#365716,#365717,#365718,
#365719,#365720,#365721,#365722,#365723,#365724,#365725,#365726,#365727,
#365728,#365729,#365730,#365731,#365732,#365733,#365734,#365735,#365736,
#365737,#365738,#365739,#365740,#365741,#365742,#365743,#365744,#365745,
#365746,#365747,#365748,#365749,#365750,#365751,#365752,#365753,#365754,
#365755,#365756,#365757,#365758,#365759,#365760,#365761,#365762,#365763,
#365764,#365765,#365766,#365767,#365768,#365769,#365770,#365771,#365772,
#365773,#365774,#365775),(#365776,#365777,#365778,#365779,#365780,#365781,
#365782,#365783,#365784,#365785,#365786,#365787,#365788,#365789,#365790,
#365791,#365792,#365793,#365794,#365795,#365796,#365797,#365798,#365799,
#365800,#365801,#365802,#365803,#365804,#365805,#365806,#365807,#365808,
#365809,#365810,#365811,#365812,#365813,#365814,#365815,#365816,#365817,
#365818,#365819,#365820,#365821,#365822,#365823,#365824,#365825,#365826,
#365827,#365828,#365829,#365830,#365831,#365832,#365833,#365834,#365835,
#365836,#365837,#365838,#365839,#365840,#365841,#365842,#365843,#365844,
#365845,#365846,#365847,#365848,#365849,#365850,#365851,#365852,#365853,
#365854,#365855,#365856,#365857,#365858,#365859,#365860,#365861,#365862,
#365863,#365864,#365865,#365866,#365867,#365868,#365869,#365870,#365871,
#365872,#365873,#365874),(#365875,#365876,#365877,#365878,#365879,#365880,
#365881,#365882,#365883,#365884,#365885,#365886,#365887,#365888,#365889,
#365890,#365891,#365892,#365893,#365894,#365895,#365896,#365897,#365898,
#365899,#365900,#365901,#365902,#365903,#365904,#365905,#365906,#365907,
#365908,#365909,#365910,#365911,#365912,#365913,#365914,#365915,#365916,
#365917,#365918,#365919,#365920,#365921,#365922,#365923,#365924,#365925,
#365926,#365927,#365928,#365929,#365930,#365931,#365932,#365933,#365934,
#365935,#365936,#365937,#365938,#365939,#365940,#365941,#365942,#365943,
#365944,#365945,#365946,#365947,#365948,#365949,#365950,#365951,#365952,
#365953,#365954,#365955,#365956,#365957,#365958,#365959,#365960,#365961,
#365962,#365963,#365964,#365965,#365966,#365967,#365968,#365969,#365970,
#365971,#365972,#365973)),.UNSPECIFIED.,.T.,.F.,.F.)
B_SPLINE_SURFACE_WITH_KNOTS((4,3,4),(4,1,1,1,1,1,1,1,1,1,1,1,1,1,1,1,1,
1,1,1,1,1,1,1,1,1,1,1,1,1,1,1,1,1,1,1,1,1,1,1,1,1,1,1,1,1,1,1,1,1,1,1,1,
1,1,1,1,1,1,1,1,1,1,1,1,1,1,1,1,1,1,1,1,1,1,1,1,1,1,1,1,1,1,1,1,1,1,1,1,
1,1,1,1,1,1,1,4),(0.,0.5,1.),(0.,0.0104467457848562,0.0208697051534179,
0.0312830741812588,0.0417059245369557,0.0521151844214314,0.0625350854994869,
0.072955523619078,0.0833651614361216,0.093785355257659,0.104205506224069,
0.114615259182489,0.125035444608255,0.135455580151817,0.145865343296126,
0.156285526040368,0.166705661591602,0.177115425208493,0.187535607700786,
0.197955743339009,0.208365506953668,0.218785689432554,0.229205825080053,
0.239615588692213,0.250035771170918,0.260455906818944,0.270865670430874,
0.281285852909622,0.291705988557657,0.302115752169577,0.312535934648329,
0.322956070296362,0.333365833908282,0.343786016387035,0.354206152035067,
0.364615915646988,0.375036098125741,0.385456233773773,0.395865997385694,
0.406286179864446,0.416706315512479,0.427116079124399,0.437536261603152,
0.447956397251184,0.458366160863105,0.468786343341857,0.47920647898989,
0.48961624260181,0.500036425080563,0.510456560728595,0.520866324340516,
0.531286506819269,0.541706642467301,0.552116406079222,0.562536588557974,
0.572956724206007,0.583366487817927,0.59378667029668,0.604206805944712,
0.614616569556633,0.625036752035385,0.635456887683418,0.645866651295338,
0.656286833774091,0.666706969422123,0.677116733034044,0.687536915512797,
0.697957051160829,0.708366814772749,0.718786997251504,0.729207132899531,
0.739616896511461,0.750037078990207,0.760457214638192,0.770866978250353,
0.781287160728572,0.791707296376735,0.802117059991444,0.812537242460403,
0.822957378121908,0.833367141740239,0.843787324122365,0.85420746003523,
0.864617223206175,0.875037405580635,0.885457544175532,0.895867297492078,
0.906287495257385,0.916707642366043,0.927117283641006,0.937537767903979,
0.947957624414904,0.958366904818021,0.968789794286159,0.979203137018726,
0.989626134310512,1.),.UNSPECIFIED.)
GEOMETRIC_REPRESENTATION_ITEM()
RATIONAL_B_SPLINE_SURFACE(((1.,1.,1.,1.,1.,1.,1.,1.,1.,1.,1.,1.,1.,1.,1.,
1.,1.,1.,1.,1.,1.,1.,1.,1.,1.,1.,1.,1.,1.,1.,1.,1.,1.,1.,1.,1.,1.,1.,1.,
1.,1.,1.,1.,1.,1.,1.,1.,1.,1.,1.,1.,1.,1.,1.,1.,1.,1.,1.,1.,1.,1.,1.,1.,
1.,1.,1.,1.,1.,1.,1.,1.,1.,1.,1.,1.,1.,1.,1.,1.,1.,1.,1.,1.,1.,1.,1.,1.,
1.,1.,1.,1.,1.,1.,1.,1.,1.,1.,1.,1.),(0.333333333333333,0.333333333333333,
0.333333333333333,0.333333333333333,0.333333333333333,0.333333333333333,
0.333333333333333,0.333333333333333,0.333333333333333,0.333333333333333,
0.333333333333333,0.333333333333333,0.333333333333333,0.333333333333333,
0.333333333333333,0.333333333333333,0.333333333333333,0.333333333333333,
0.333333333333333,0.333333333333333,0.333333333333333,0.333333333333333,
0.333333333333333,0.333333333333333,0.333333333333333,0.333333333333333,
0.333333333333333,0.333333333333333,0.333333333333333,0.333333333333333,
0.333333333333333,0.333333333333333,0.333333333333333,0.333333333333333,
0.333333333333333,0.333333333333333,0.333333333333333,0.333333333333333,
0.333333333333333,0.333333333333333,0.333333333333333,0.333333333333333,
0.333333333333333,0.333333333333333,0.333333333333333,0.333333333333333,
0.333333333333333,0.333333333333333,0.333333333333333,0.333333333333333,
0.333333333333333,0.333333333333333,0.333333333333333,0.333333333333333,
0.333333333333333,0.333333333333333,0.333333333333333,0.333333333333333,
0.333333333333333,0.333333333333333,0.333333333333333,0.333333333333333,
0.333333333333333,0.333333333333333,0.333333333333333,0.333333333333333,
0.333333333333333,0.333333333333333,0.333333333333333,0.333333333333333,
0.333333333333333,0.333333333333333,0.333333333333333,0.333333333333333,
0.333333333333333,0.333333333333333,0.333333333333333,0.333333333333333,
0.333333333333333,0.333333333333333,0.333333333333333,0.333333333333333,
0.333333333333333,0.333333333333333,0.333333333333333,0.333333333333333,
0.333333333333333,0.333333333333333,0.333333333333333,0.333333333333333,
0.333333333333333,0.333333333333333,0.333333333333333,0.333333333333333,
0.333333333333333,0.333333333333333,0.333333333333333,0.333333333333333,
0.333333333333333),(0.333333333333333,0.333333333333333,0.333333333333333,
0.333333333333333,0.333333333333333,0.333333333333333,0.333333333333333,
0.333333333333333,0.333333333333333,0.333333333333333,0.333333333333333,
0.333333333333333,0.333333333333333,0.333333333333333,0.333333333333333,
0.333333333333333,0.333333333333333,0.333333333333333,0.333333333333333,
0.333333333333333,0.333333333333333,0.333333333333333,0.333333333333333,
0.333333333333333,0.333333333333333,0.333333333333333,0.333333333333333,
0.333333333333333,0.333333333333333,0.333333333333333,0.333333333333333,
0.333333333333333,0.333333333333333,0.333333333333333,0.333333333333333,
0.333333333333333,0.333333333333333,0.333333333333333,0.333333333333333,
0.333333333333333,0.333333333333333,0.333333333333333,0.333333333333333,
0.333333333333333,0.333333333333333,0.333333333333333,0.333333333333333,
0.333333333333333,0.333333333333333,0.333333333333333,0.333333333333333,
0.333333333333333,0.333333333333333,0.333333333333333,0.333333333333333,
0.333333333333333,0.333333333333333,0.333333333333333,0.333333333333333,
0.333333333333333,0.333333333333333,0.333333333333333,0.333333333333333,
0.333333333333333,0.333333333333333,0.333333333333333,0.333333333333333,
0.333333333333333,0.333333333333333,0.333333333333333,0.333333333333333,
0.333333333333333,0.333333333333333,0.333333333333333,0.333333333333333,
0.333333333333333,0.333333333333333,0.333333333333333,0.333333333333333,
0.333333333333333,0.333333333333333,0.333333333333333,0.333333333333333,
0.333333333333333,0.333333333333333,0.333333333333333,0.333333333333333,
0.333333333333333,0.333333333333333,0.333333333333333,0.333333333333333,
0.333333333333333,0.333333333333333,0.333333333333333,0.333333333333333,
0.333333333333333,0.333333333333333,0.333333333333333,0.333333333333333),
(1.,1.,1.,1.,1.,1.,1.,1.,1.,1.,1.,1.,1.,1.,1.,1.,1.,1.,1.,1.,1.,1.,1.,1.,
1.,1.,1.,1.,1.,1.,1.,1.,1.,1.,1.,1.,1.,1.,1.,1.,1.,1.,1.,1.,1.,1.,1.,1.,
1.,1.,1.,1.,1.,1.,1.,1.,1.,1.,1.,1.,1.,1.,1.,1.,1.,1.,1.,1.,1.,1.,1.,1.,
1.,1.,1.,1.,1.,1.,1.,1.,1.,1.,1.,1.,1.,1.,1.,1.,1.,1.,1.,1.,1.,1.,1.,1.,
1.,1.,1.),(0.333333333333333,0.333333333333333,0.333333333333333,0.333333333333333,
0.333333333333333,0.333333333333333,0.333333333333333,0.333333333333333,
0.333333333333333,0.333333333333333,0.333333333333333,0.333333333333333,
0.333333333333333,0.333333333333333,0.333333333333333,0.333333333333333,
0.333333333333333,0.333333333333333,0.333333333333333,0.333333333333333,
0.333333333333333,0.333333333333333,0.333333333333333,0.333333333333333,
0.333333333333333,0.333333333333333,0.333333333333333,0.333333333333333,
0.333333333333333,0.333333333333333,0.333333333333333,0.333333333333333,
0.333333333333333,0.333333333333333,0.333333333333333,0.333333333333333,
0.333333333333333,0.333333333333333,0.333333333333333,0.333333333333333,
0.333333333333333,0.333333333333333,0.333333333333333,0.333333333333333,
0.333333333333333,0.333333333333333,0.333333333333333,0.333333333333333,
0.333333333333333,0.333333333333333,0.333333333333333,0.333333333333333,
0.333333333333333,0.333333333333333,0.333333333333333,0.333333333333333,
0.333333333333333,0.333333333333333,0.333333333333333,0.333333333333333,
0.333333333333333,0.333333333333333,0.333333333333333,0.333333333333333,
0.333333333333333,0.333333333333333,0.333333333333333,0.333333333333333,
0.333333333333333,0.333333333333333,0.333333333333333,0.333333333333333,
0.333333333333333,0.333333333333333,0.333333333333333,0.333333333333333,
0.333333333333333,0.333333333333333,0.333333333333333,0.333333333333333,
0.333333333333333,0.333333333333333,0.333333333333333,0.333333333333333,
0.333333333333333,0.333333333333333,0.333333333333333,0.333333333333333,
0.333333333333333,0.333333333333333,0.333333333333333,0.333333333333333,
0.333333333333333,0.333333333333333,0.333333333333333,0.333333333333333,
0.333333333333333,0.333333333333333,0.333333333333333),(0.333333333333333,
0.333333333333333,0.333333333333333,0.333333333333333,0.333333333333333,
0.333333333333333,0.333333333333333,0.333333333333333,0.333333333333333,
0.333333333333333,0.333333333333333,0.333333333333333,0.333333333333333,
0.333333333333333,0.333333333333333,0.333333333333333,0.333333333333333,
0.333333333333333,0.333333333333333,0.333333333333333,0.333333333333333,
0.333333333333333,0.333333333333333,0.333333333333333,0.333333333333333,
0.333333333333333,0.333333333333333,0.333333333333333,0.333333333333333,
0.333333333333333,0.333333333333333,0.333333333333333,0.333333333333333,
0.333333333333333,0.333333333333333,0.333333333333333,0.333333333333333,
0.333333333333333,0.333333333333333,0.333333333333333,0.333333333333333,
0.333333333333333,0.333333333333333,0.333333333333333,0.333333333333333,
0.333333333333333,0.333333333333333,0.333333333333333,0.333333333333333,
0.333333333333333,0.333333333333333,0.333333333333333,0.333333333333333,
0.333333333333333,0.333333333333333,0.333333333333333,0.333333333333333,
0.333333333333333,0.333333333333333,0.333333333333333,0.333333333333333,
0.333333333333333,0.333333333333333,0.333333333333333,0.333333333333333,
0.333333333333333,0.333333333333333,0.333333333333333,0.333333333333333,
0.333333333333333,0.333333333333333,0.333333333333333,0.333333333333333,
0.333333333333333,0.333333333333333,0.333333333333333,0.333333333333333,
0.333333333333333,0.333333333333333,0.333333333333333,0.333333333333333,
0.333333333333333,0.333333333333333,0.333333333333333,0.333333333333333,
0.333333333333333,0.333333333333333,0.333333333333333,0.333333333333333,
0.333333333333333,0.333333333333333,0.333333333333333,0.333333333333333,
0.333333333333333,0.333333333333333,0.333333333333333,0.333333333333333,
0.333333333333333,0.333333333333333),(1.,1.,1.,1.,1.,1.,1.,1.,1.,1.,1.,
1.,1.,1.,1.,1.,1.,1.,1.,1.,1.,1.,1.,1.,1.,1.,1.,1.,1.,1.,1.,1.,1.,1.,1.,
1.,1.,1.,1.,1.,1.,1.,1.,1.,1.,1.,1.,1.,1.,1.,1.,1.,1.,1.,1.,1.,1.,1.,1.,
1.,1.,1.,1.,1.,1.,1.,1.,1.,1.,1.,1.,1.,1.,1.,1.,1.,1.,1.,1.,1.,1.,1.,1.,
1.,1.,1.,1.,1.,1.,1.,1.,1.,1.,1.,1.,1.,1.,1.,1.)))
REPRESENTATION_ITEM('')
SURFACE()
);
#2314=(
BOUNDED_SURFACE()
B_SPLINE_SURFACE(3,3,((#365979,#365980,#365981,#365982,#365983,#365984,
#365985,#365986,#365987,#365988,#365989,#365990,#365991,#365992,#365993,
#365994,#365995,#365996,#365997,#365998,#365999,#366000,#366001,#366002,
#366003,#366004,#366005,#366006,#366007),(#366008,#366009,#366010,#366011,
#366012,#366013,#366014,#366015,#366016,#366017,#366018,#366019,#366020,
#366021,#366022,#366023,#366024,#366025,#366026,#366027,#366028,#366029,
#366030,#366031,#366032,#366033,#366034,#366035,#366036),(#366037,#366038,
#366039,#366040,#366041,#366042,#366043,#366044,#366045,#366046,#366047,
#366048,#366049,#366050,#366051,#366052,#366053,#366054,#366055,#366056,
#366057,#366058,#366059,#366060,#366061,#366062,#366063,#366064,#366065),
(#366066,#366067,#366068,#366069,#366070,#366071,#366072,#366073,#366074,
#366075,#366076,#366077,#366078,#366079,#366080,#366081,#366082,#366083,
#366084,#366085,#366086,#366087,#366088,#366089,#366090,#366091,#366092,
#366093,#366094),(#366095,#366096,#366097,#366098,#366099,#366100,#366101,
#366102,#366103,#366104,#366105,#366106,#366107,#366108,#366109,#366110,
#366111,#366112,#366113,#366114,#366115,#366116,#366117,#366118,#366119,
#366120,#366121,#366122,#366123),(#366124,#366125,#366126,#366127,#366128,
#366129,#366130,#366131,#366132,#366133,#366134,#366135,#366136,#366137,
#366138,#366139,#366140,#366141,#366142,#366143,#366144,#366145,#366146,
#366147,#366148,#366149,#366150,#366151,#366152),(#366153,#366154,#366155,
#366156,#366157,#366158,#366159,#366160,#366161,#366162,#366163,#366164,
#366165,#366166,#366167,#366168,#366169,#366170,#366171,#366172,#366173,
#366174,#366175,#366176,#366177,#366178,#366179,#366180,#366181)),
 .UNSPECIFIED.,.T.,.F.,.F.)
B_SPLINE_SURFACE_WITH_KNOTS((4,3,4),(4,1,1,1,1,1,1,1,1,1,1,1,1,1,1,1,1,
1,1,1,1,1,1,1,1,1,4),(0.,0.5,1.),(0.,0.0310703336761616,0.0624385278003938,
0.0937144048499659,0.124978469089869,0.166663774179581,0.208294236860357,
0.249966520356582,0.291641529650434,0.3332733240007,0.374947073344913,0.416620808022619,
0.458253030541402,0.499926784452264,0.54160045129851,0.583232674441905,
0.624906496125386,0.666580158626562,0.708211959489969,0.749887054558503,
0.791559255246094,0.833189756589646,0.87487513422873,0.906139159779086,
0.937415106668169,0.968783217665703,1.),.UNSPECIFIED.)
GEOMETRIC_REPRESENTATION_ITEM()
RATIONAL_B_SPLINE_SURFACE(((1.,1.,1.,1.,1.,1.,1.,1.,1.,1.,1.,1.,1.,1.,1.,
1.,1.,1.,1.,1.,1.,1.,1.,1.,1.,1.,1.,1.,1.),(0.333333333333333,0.333333333333333,
0.333333333333334,0.333333333333333,0.333333333333333,0.333333333333333,
0.333333333333333,0.333333333333333,0.333333333333333,0.333333333333333,
0.333333333333333,0.333333333333333,0.333333333333334,0.333333333333333,
0.333333333333333,0.333333333333333,0.333333333333333,0.333333333333333,
0.333333333333333,0.333333333333333,0.333333333333333,0.333333333333333,
0.333333333333333,0.333333333333333,0.333333333333333,0.333333333333333,
0.333333333333333,0.333333333333333,0.333333333333333),(0.333333333333333,
0.333333333333333,0.333333333333334,0.333333333333333,0.333333333333333,
0.333333333333333,0.333333333333333,0.333333333333333,0.333333333333333,
0.333333333333333,0.333333333333333,0.333333333333333,0.333333333333334,
0.333333333333333,0.333333333333333,0.333333333333333,0.333333333333333,
0.333333333333333,0.333333333333333,0.333333333333333,0.333333333333333,
0.333333333333333,0.333333333333333,0.333333333333333,0.333333333333333,
0.333333333333333,0.333333333333333,0.333333333333333,0.333333333333333),
(1.,1.,1.,1.,1.,1.,1.,1.,1.,1.,1.,1.,1.,1.,1.,1.,1.,1.,1.,1.,1.,1.,1.,1.,
1.,1.,1.,1.,1.),(0.333333333333333,0.333333333333333,0.333333333333334,
0.333333333333333,0.333333333333333,0.333333333333333,0.333333333333333,
0.333333333333333,0.333333333333333,0.333333333333333,0.333333333333333,
0.333333333333333,0.333333333333334,0.333333333333333,0.333333333333333,
0.333333333333333,0.333333333333333,0.333333333333333,0.333333333333333,
0.333333333333333,0.333333333333333,0.333333333333333,0.333333333333333,
0.333333333333333,0.333333333333333,0.333333333333333,0.333333333333333,
0.333333333333333,0.333333333333333),(0.333333333333333,0.333333333333333,
0.333333333333334,0.333333333333333,0.333333333333333,0.333333333333333,
0.333333333333333,0.333333333333333,0.333333333333333,0.333333333333333,
0.333333333333333,0.333333333333333,0.333333333333334,0.333333333333333,
0.333333333333333,0.333333333333333,0.333333333333333,0.333333333333333,
0.333333333333333,0.333333333333333,0.333333333333333,0.333333333333333,
0.333333333333333,0.333333333333333,0.333333333333333,0.333333333333333,
0.333333333333333,0.333333333333333,0.333333333333333),(1.,1.,1.,1.,1.,
1.,1.,1.,1.,1.,1.,1.,1.,1.,1.,1.,1.,1.,1.,1.,1.,1.,1.,1.,1.,1.,1.,1.,1.)))
REPRESENTATION_ITEM('')
SURFACE()
);
#4415=SHAPE_REPRESENTATION_RELATIONSHIP('SRR','None',#459341,#4436);
#4436=ADVANCED_BREP_SHAPE_REPRESENTATION('',(#4468),#459230);
#4468=MANIFOLD_SOLID_BREP('Body1',#94646);
#4588=STYLED_ITEM('',(#459526),#4468);
#5695=PLANE('',#99164);
#5696=PLANE('',#99167);
#8400=FACE_OUTER_BOUND('',#14308,.T.);
#8401=FACE_OUTER_BOUND('',#14309,.T.);
#8402=FACE_OUTER_BOUND('',#14310,.T.);
#8403=FACE_OUTER_BOUND('',#14311,.T.);
#8404=FACE_OUTER_BOUND('',#14312,.T.);
#8405=FACE_OUTER_BOUND('',#14313,.T.);
#8406=FACE_OUTER_BOUND('',#14314,.T.);
#8407=FACE_OUTER_BOUND('',#14315,.T.);
#14308=EDGE_LOOP('',(#69238,#69239,#69240,#69241,#69242));
#14309=EDGE_LOOP('',(#69243,#69244,#69245,#69246,#69247,#69248));
#14310=EDGE_LOOP('',(#69249,#69250,#69251,#69252,#69253));
#14311=EDGE_LOOP('',(#69254,#69255,#69256,#69257,#69258));
#14312=EDGE_LOOP('',(#69259,#69260));
#14313=EDGE_LOOP('',(#69261,#69262,#69263,#69264,#69265,#69266));
#14314=EDGE_LOOP('',(#69267,#69268));
#14315=EDGE_LOOP('',(#69269,#69270,#69271,#69272,#69273));
#24631=B_SPLINE_CURVE_WITH_KNOTS('',3,(#363851,#363852,#363853,#363854,
#363855,#363856,#363857,#363858,#363859,#363860,#363861,#363862,#363863,
#363864,#363865,#363866,#363867,#363868,#363869,#363870,#363871,#363872,
#363873,#363874,#363875,#363876,#363877,#363878,#363879),.UNSPECIFIED.,
 .F.,.F.,(4,1,1,1,1,1,1,1,1,1,1,1,1,1,1,1,1,1,1,1,1,1,1,1,1,1,4),(0.,0.0310703336761616,
0.0624385278003938,0.0937144048499659,0.124978469089869,0.166663774179581,
0.208294236860357,0.249966520356582,0.291641529650434,0.3332733240007,0.374947073344913,
0.416620808022619,0.458253030541402,0.499926784452264,0.54160045129851,
0.583232674441905,0.624906496125386,0.666580158626562,0.708211959489969,
0.749887054558503,0.791559255246094,0.833189756589646,0.87487513422873,
0.906139159779086,0.937415106668169,0.968783217665703,1.),.UNSPECIFIED.);
#24632=B_SPLINE_CURVE_WITH_KNOTS('',3,(#363883,#363884,#363885,#363886,
#363887,#363888,#363889,#363890,#363891,#363892,#363893,#363894,#363895,
#363896,#363897,#363898,#363899,#363900,#363901,#363902,#363903,#363904,
#363905,#363906,#363907,#363908,#363909,#363910,#363911),.UNSPECIFIED.,
 .F.,.F.,(4,1,1,1,1,1,1,1,1,1,1,1,1,1,1,1,1,1,1,1,1,1,1,1,1,1,4),(0.,0.0310703336761616,
0.0624385278003938,0.0937144048499659,0.124978469089869,0.166663774179581,
0.208294236860357,0.249966520356582,0.291641529650434,0.3332733240007,0.374947073344913,
0.416620808022619,0.458253030541402,0.499926784452264,0.54160045129851,
0.583232674441905,0.624906496125386,0.666580158626562,0.708211959489969,
0.749887054558503,0.791559255246094,0.833189756589646,0.87487513422873,
0.906139159779086,0.937415106668169,0.968783217665703,1.),.UNSPECIFIED.);
#24633=B_SPLINE_CURVE_WITH_KNOTS('',3,(#364611,#364612,#364613,#364614,
#364615,#364616,#364617,#364618,#364619,#364620,#364621,#364622,#364623,
#364624,#364625,#364626,#364627,#364628,#364629,#364630,#364631,#364632,
#364633,#364634,#364635,#364636,#364637,#364638,#364639,#364640,#364641,
#364642,#364643,#364644,#364645,#364646,#364647,#364648,#364649,#364650,
#364651,#364652,#364653,#364654,#364655,#364656,#364657,#364658,#364659,
#364660,#364661,#364662,#364663,#364664,#364665,#364666,#364667,#364668,
#364669,#364670,#364671,#364672,#364673,#364674,#364675,#364676,#364677,
#364678,#364679,#364680,#364681,#364682,#364683,#364684,#364685,#364686,
#364687,#364688,#364689,#364690,#364691,#364692,#364693,#364694,#364695,
#364696,#364697,#364698,#364699,#364700,#364701,#364702,#364703,#364704,
#364705,#364706,#364707,#364708,#364709),.UNSPECIFIED.,.F.,.F.,(4,1,1,1,
1,1,1,1,1,1,1,1,1,1,1,1,1,1,1,1,1,1,1,1,1,1,1,1,1,1,1,1,1,1,1,1,1,1,1,1,
1,1,1,1,1,1,1,1,1,1,1,1,1,1,1,1,1,1,1,1,1,1,1,1,1,1,1,1,1,1,1,1,1,1,1,1,
1,1,1,1,1,1,1,1,1,1,1,1,1,1,1,1,1,1,1,1,4),(0.,0.0104467457848562,0.0208697051534179,
0.0312830741812588,0.0417059245369557,0.0521151844214314,0.0625350854994869,
0.072955523619078,0.0833651614361216,0.093785355257659,0.104205506224069,
0.114615259182489,0.125035444608255,0.135455580151817,0.145865343296126,
0.156285526040368,0.166705661591602,0.177115425208493,0.187535607700786,
0.197955743339009,0.208365506953668,0.218785689432554,0.229205825080053,
0.239615588692213,0.250035771170918,0.260455906818944,0.270865670430874,
0.281285852909622,0.291705988557657,0.302115752169577,0.312535934648329,
0.322956070296362,0.333365833908282,0.343786016387035,0.354206152035067,
0.364615915646988,0.375036098125741,0.385456233773773,0.395865997385694,
0.406286179864446,0.416706315512479,0.427116079124399,0.437536261603152,
0.447956397251184,0.458366160863105,0.468786343341857,0.47920647898989,
0.48961624260181,0.500036425080563,0.510456560728595,0.520866324340516,
0.531286506819269,0.541706642467301,0.552116406079222,0.562536588557974,
0.572956724206007,0.583366487817927,0.59378667029668,0.604206805944712,
0.614616569556633,0.625036752035385,0.635456887683418,0.645866651295338,
0.656286833774091,0.666706969422123,0.677116733034044,0.687536915512797,
0.697957051160829,0.708366814772749,0.718786997251504,0.729207132899531,
0.739616896511461,0.750037078990207,0.760457214638192,0.770866978250353,
0.781287160728572,0.791707296376735,0.802117059991444,0.812537242460403,
0.822957378121908,0.833367141740239,0.843787324122365,0.85420746003523,
0.864617223206175,0.875037405580635,0.885457544175532,0.895867297492078,
0.906287495257385,0.916707642366043,0.927117283641006,0.937537767903979,
0.947957624414904,0.958366904818021,0.968789794286159,0.979203137018726,
0.989626134310512,1.),.UNSPECIFIED.);
#24634=B_SPLINE_CURVE_WITH_KNOTS('',3,(#364710,#364711,#364712,#364713,
#364714,#364715,#364716,#364717,#364718,#364719,#364720,#364721,#364722,
#364723,#364724,#364725,#364726,#364727,#364728,#364729,#364730,#364731,
#364732,#364733,#364734,#364735,#364736,#364737,#364738,#364739,#364740,
#364741,#364742,#364743,#364744,#364745,#364746,#364747,#364748,#364749,
#364750,#364751,#364752,#364753,#364754,#364755,#364756,#364757,#364758,
#364759,#364760,#364761,#364762,#364763,#364764,#364765,#364766,#364767,
#364768,#364769,#364770,#364771,#364772,#364773,#364774,#364775,#364776,
#364777,#364778,#364779,#364780,#364781,#364782,#364783,#364784,#364785,
#364786,#364787,#364788,#364789,#364790,#364791,#364792,#364793,#364794,
#364795,#364796,#364797,#364798,#364799,#364800,#364801,#364802,#364803,
#364804,#364805,#364806,#364807,#364808),.UNSPECIFIED.,.F.,.F.,(4,1,1,1,
1,1,1,1,1,1,1,1,1,1,1,1,1,1,1,1,1,1,1,1,1,1,1,1,1,1,1,1,1,1,1,1,1,1,1,1,
1,1,1,1,1,1,1,1,1,1,1,1,1,1,1,1,1,1,1,1,1,1,1,1,1,1,1,1,1,1,1,1,1,1,1,1,
1,1,1,1,1,1,1,1,1,1,1,1,1,1,1,1,1,1,1,1,4),(0.,0.0104467457848562,0.0208697051534179,
0.0312830741812588,0.0417059245369557,0.0521151844214314,0.0625350854994869,
0.072955523619078,0.0833651614361216,0.093785355257659,0.104205506224069,
0.114615259182489,0.125035444608255,0.135455580151817,0.145865343296126,
0.156285526040368,0.166705661591602,0.177115425208493,0.187535607700786,
0.197955743339009,0.208365506953668,0.218785689432554,0.229205825080053,
0.239615588692213,0.250035771170918,0.260455906818944,0.270865670430874,
0.281285852909622,0.291705988557657,0.302115752169577,0.312535934648329,
0.322956070296362,0.333365833908282,0.343786016387035,0.354206152035067,
0.364615915646988,0.375036098125741,0.385456233773773,0.395865997385694,
0.406286179864446,0.416706315512479,0.427116079124399,0.437536261603152,
0.447956397251184,0.458366160863105,0.468786343341857,0.47920647898989,
0.48961624260181,0.500036425080563,0.510456560728595,0.520866324340516,
0.531286506819269,0.541706642467301,0.552116406079222,0.562536588557974,
0.572956724206007,0.583366487817927,0.59378667029668,0.604206805944712,
0.614616569556633,0.625036752035385,0.635456887683418,0.645866651295338,
0.656286833774091,0.666706969422123,0.677116733034044,0.687536915512797,
0.697957051160829,0.708366814772749,0.718786997251504,0.729207132899531,
0.739616896511461,0.750037078990207,0.760457214638192,0.770866978250353,
0.781287160728572,0.791707296376735,0.802117059991444,0.812537242460403,
0.822957378121908,0.833367141740239,0.843787324122365,0.85420746003523,
0.864617223206175,0.875037405580635,0.885457544175532,0.895867297492078,
0.906287495257385,0.916707642366043,0.927117283641006,0.937537767903979,
0.947957624414904,0.958366904818021,0.968789794286159,0.979203137018726,
0.989626134310512,1.),.UNSPECIFIED.);
#24635=B_SPLINE_CURVE_WITH_KNOTS('',3,(#365015,#365016,#365017,#365018,
#365019,#365020,#365021,#365022,#365023,#365024,#365025,#365026,#365027,
#365028,#365029,#365030,#365031,#365032,#365033,#365034,#365035,#365036,
#365037,#365038,#365039,#365040,#365041,#365042,#365043),.UNSPECIFIED.,
 .F.,.F.,(4,1,1,1,1,1,1,1,1,1,1,1,1,1,1,1,1,1,1,1,1,1,1,1,1,1,4),(0.,0.0311997468912562,
0.0625509890871527,0.0938098447846757,0.1250568872711,0.166719530856106,
0.208327420639085,0.249977065870109,0.291629399375196,0.333238604634684,
0.374889730322128,0.41654078485731,0.458150415717,0.499801548056339,0.541452534012182,
0.583062165488229,0.624713366295055,0.666364346005318,0.707973557473876,
0.749626035232519,0.791275541260273,0.832883464833855,0.874546235186119,
0.905793212129613,0.937052173453026,0.968403278656631,1.),.UNSPECIFIED.);
#24636=B_SPLINE_CURVE_WITH_KNOTS('',3,(#365044,#365045,#365046,#365047,
#365048,#365049,#365050,#365051,#365052,#365053,#365054,#365055,#365056,
#365057,#365058,#365059,#365060,#365061,#365062,#365063,#365064,#365065,
#365066,#365067,#365068,#365069,#365070,#365071,#365072),.UNSPECIFIED.,
 .F.,.F.,(4,1,1,1,1,1,1,1,1,1,1,1,1,1,1,1,1,1,1,1,1,1,1,1,1,1,4),(0.,0.0311997468912562,
0.0625509890871527,0.0938098447846757,0.1250568872711,0.166719530856106,
0.208327420639085,0.249977065870109,0.291629399375196,0.333238604634684,
0.374889730322128,0.41654078485731,0.458150415717,0.499801548056339,0.541452534012182,
0.583062165488229,0.624713366295055,0.666364346005318,0.707973557473876,
0.749626035232519,0.791275541260273,0.832883464833855,0.874546235186119,
0.905793212129613,0.937052173453026,0.968403278656631,1.),.UNSPECIFIED.);
#38281=VERTEX_POINT('',#363847);
#38282=VERTEX_POINT('',#363848);
#38283=VERTEX_POINT('',#363850);
#38284=VERTEX_POINT('',#363880);
#38285=VERTEX_POINT('',#363882);
#38286=VERTEX_POINT('',#364606);
#38287=VERTEX_POINT('',#364607);
#38288=VERTEX_POINT('',#364609);
#38289=VERTEX_POINT('',#365012);
#38290=VERTEX_POINT('',#365013);
#38291=VERTEX_POINT('',#365277);
#38292=VERTEX_POINT('',#365974);
#49121=EDGE_CURVE('',#38281,#38282,#186,.T.);
#49122=EDGE_CURVE('',#38281,#38283,#24631,.T.);
#49123=EDGE_CURVE('',#38284,#38283,#187,.T.);
#49124=EDGE_CURVE('',#38285,#38284,#24632,.T.);
#49125=EDGE_CURVE('',#38282,#38285,#188,.T.);
#49126=EDGE_CURVE('',#38286,#38287,#189,.T.);
#49127=EDGE_CURVE('',#38287,#38288,#190,.T.);
#49128=EDGE_CURVE('',#38288,#38281,#24633,.T.);
#49129=EDGE_CURVE('',#38286,#38285,#24634,.T.);
#49130=EDGE_CURVE('',#38289,#38290,#191,.T.);
#49131=EDGE_CURVE('',#38289,#38288,#24635,.T.);
#49132=EDGE_CURVE('',#38290,#38286,#24636,.T.);
#49133=EDGE_CURVE('',#38290,#38289,#192,.T.);
#49134=EDGE_CURVE('',#38291,#38286,#193,.T.);
#49135=EDGE_CURVE('',#38288,#38291,#194,.T.);
#49136=EDGE_CURVE('',#38285,#38292,#195,.T.);
#49137=EDGE_CURVE('',#38292,#38281,#196,.T.);
#49138=EDGE_CURVE('',#38283,#38284,#197,.T.);
#69238=ORIENTED_EDGE('',*,*,#49121,.F.);
#69239=ORIENTED_EDGE('',*,*,#49122,.T.);
#69240=ORIENTED_EDGE('',*,*,#49123,.F.);
#69241=ORIENTED_EDGE('',*,*,#49124,.F.);
#69242=ORIENTED_EDGE('',*,*,#49125,.F.);
#69243=ORIENTED_EDGE('',*,*,#49126,.T.);
#69244=ORIENTED_EDGE('',*,*,#49127,.T.);
#69245=ORIENTED_EDGE('',*,*,#49128,.T.);
#69246=ORIENTED_EDGE('',*,*,#49121,.T.);
#69247=ORIENTED_EDGE('',*,*,#49125,.T.);
#69248=ORIENTED_EDGE('',*,*,#49129,.F.);
#69249=ORIENTED_EDGE('',*,*,#49130,.F.);
#69250=ORIENTED_EDGE('',*,*,#49131,.T.);
#69251=ORIENTED_EDGE('',*,*,#49127,.F.);
#69252=ORIENTED_EDGE('',*,*,#49126,.F.);
#69253=ORIENTED_EDGE('',*,*,#49132,.F.);
#69254=ORIENTED_EDGE('',*,*,#49131,.F.);
#69255=ORIENTED_EDGE('',*,*,#49133,.F.);
#69256=ORIENTED_EDGE('',*,*,#49132,.T.);
#69257=ORIENTED_EDGE('',*,*,#49134,.F.);
#69258=ORIENTED_EDGE('',*,*,#49135,.F.);
#69259=ORIENTED_EDGE('',*,*,#49133,.T.);
#69260=ORIENTED_EDGE('',*,*,#49130,.T.);
#69261=ORIENTED_EDGE('',*,*,#49128,.F.);
#69262=ORIENTED_EDGE('',*,*,#49135,.T.);
#69263=ORIENTED_EDGE('',*,*,#49134,.T.);
#69264=ORIENTED_EDGE('',*,*,#49129,.T.);
#69265=ORIENTED_EDGE('',*,*,#49136,.T.);
#69266=ORIENTED_EDGE('',*,*,#49137,.T.);
#69267=ORIENTED_EDGE('',*,*,#49123,.T.);
#69268=ORIENTED_EDGE('',*,*,#49138,.T.);
#69269=ORIENTED_EDGE('',*,*,#49122,.F.);
#69270=ORIENTED_EDGE('',*,*,#49137,.F.);
#69271=ORIENTED_EDGE('',*,*,#49136,.F.);
#69272=ORIENTED_EDGE('',*,*,#49124,.T.);
#69273=ORIENTED_EDGE('',*,*,#49138,.F.);
#90864=ADVANCED_FACE('',(#8400),#2309,.F.);
#90865=ADVANCED_FACE('',(#8401),#2310,.T.);
#90866=ADVANCED_FACE('',(#8402),#2311,.F.);
#90867=ADVANCED_FACE('',(#8403),#2312,.F.);
#90868=ADVANCED_FACE('',(#8404),#5695,.T.);
#90869=ADVANCED_FACE('',(#8405),#2313,.T.);
#90870=ADVANCED_FACE('',(#8406),#5696,.T.);
#90871=ADVANCED_FACE('',(#8407),#2314,.F.);
#94646=CLOSED_SHELL('',(#90864,#90865,#90866,#90867,#90868,#90869,#90870,
#90871));
#99154=AXIS2_PLACEMENT_3D('',#363643,#116003,#116004);
#99155=AXIS2_PLACEMENT_3D('',#363849,#116005,#116006);
#99156=AXIS2_PLACEMENT_3D('',#363881,#116007,#116008);
#99157=AXIS2_PLACEMENT_3D('',#363912,#116009,#116010);
#99158=AXIS2_PLACEMENT_3D('',#364608,#116011,#116012);
#99159=AXIS2_PLACEMENT_3D('',#364610,#116013,#116014);
#99160=AXIS2_PLACEMENT_3D('',#365014,#116015,#116016);
#99161=AXIS2_PLACEMENT_3D('',#365276,#116017,#116018);
#99162=AXIS2_PLACEMENT_3D('',#365278,#116019,#116020);
#99163=AXIS2_PLACEMENT_3D('',#365279,#116021,#116022);
#99164=AXIS2_PLACEMENT_3D('',#365280,#116023,#116024);
#99165=AXIS2_PLACEMENT_3D('',#365975,#116025,#116026);
#99166=AXIS2_PLACEMENT_3D('',#365976,#116027,#116028);
#99167=AXIS2_PLACEMENT_3D('',#365977,#116029,#116030);
#99168=AXIS2_PLACEMENT_3D('',#365978,#116031,#116032);
#116003=DIRECTION('axis',(0.,0.,1.));
#116004=DIRECTION('refdir',(1.,0.,0.));
#116005=DIRECTION('center_axis',(1.90014037850669E-13,0.994089659369792,
0.108562190167897));
#116006=DIRECTION('ref_axis',(0.999999999984429,-6.05836258509456E-7,5.54756097781441E-6));
#116007=DIRECTION('center_axis',(-1.04862710274864E-14,-0.997667534637082,
-0.0682604595001084));
#116008=DIRECTION('ref_axis',(0.99999999997237,-5.07429128929804E-7,7.41638074638744E-6));
#116009=DIRECTION('center_axis',(1.90014037850669E-13,0.994089659369792,
0.108562190167897));
#116010=DIRECTION('ref_axis',(0.999999999984429,-6.05836258509456E-7,5.54756097781441E-6));
#116011=DIRECTION('center_axis',(4.15449470707835E-15,-0.994089659369792,
-0.108562190167898));
#116012=DIRECTION('ref_axis',(0.999999999999024,-1.5165736758839E-7,1.38870655435557E-6));
#116013=DIRECTION('center_axis',(4.15449470707835E-15,-0.994089659369792,
-0.108562190167898));
#116014=DIRECTION('ref_axis',(0.999999999999024,-1.5165736758839E-7,1.38870655435557E-6));
#116015=DIRECTION('center_axis',(0.,1.,0.));
#116016=DIRECTION('ref_axis',(1.,0.,0.));
#116017=DIRECTION('center_axis',(0.,1.,0.));
#116018=DIRECTION('ref_axis',(1.,0.,0.));
#116019=DIRECTION('center_axis',(4.15449470707834E-15,-0.994089659369792,
-0.108562190167898));
#116020=DIRECTION('ref_axis',(0.999999999999024,-1.51657367553393E-7,1.3887065540351E-6));
#116021=DIRECTION('center_axis',(4.15449470707834E-15,-0.994089659369792,
-0.108562190167898));
#116022=DIRECTION('ref_axis',(0.999999999999024,-1.51657367553393E-7,1.3887065540351E-6));
#116023=DIRECTION('center_axis',(0.,1.,0.));
#116024=DIRECTION('ref_axis',(0.,0.,1.));
#116025=DIRECTION('center_axis',(-1.41956054810603E-13,0.994089659369792,
0.108562190167897));
#116026=DIRECTION('ref_axis',(0.999999999984429,-6.05835921327016E-7,5.54756094815878E-6));
#116027=DIRECTION('center_axis',(-1.41956054810603E-13,0.994089659369792,
0.108562190167897));
#116028=DIRECTION('ref_axis',(0.999999999984429,-6.05835921327016E-7,5.54756094815878E-6));
#116029=DIRECTION('center_axis',(-1.05710970162048E-14,-0.997667534637082,
-0.0682604595001086));
#116030=DIRECTION('ref_axis',(0.,0.0682604595001086,-0.997667534637082));
#116031=DIRECTION('center_axis',(-1.06920965951746E-14,-0.997667534637082,
-0.0682604595001082));
#116032=DIRECTION('ref_axis',(0.99999999997237,-5.07429130466677E-7,7.41638076583464E-6));
#363643=CARTESIAN_POINT('',(0.,0.,0.));
#363644=CARTESIAN_POINT('Ctrl Pts',(2.00016367750204,-0.0349606549171534,
-7.37954989315335));
#363645=CARTESIAN_POINT('Ctrl Pts',(2.00016367750204,-0.165462727384539,
-7.38526442622049));
#363646=CARTESIAN_POINT('Ctrl Pts',(1.96855967425598,-0.409173319918984,
-7.39995586097472));
#363647=CARTESIAN_POINT('Ctrl Pts',(1.85189486927969,-0.792213245836797,
-7.42009815347362));
#363648=CARTESIAN_POINT('Ctrl Pts',(1.6613582879716,-1.13645205609876,-7.44086906835104));
#363649=CARTESIAN_POINT('Ctrl Pts',(1.37992038202068,-1.47263550497672,
-7.46380724865708));
#363650=CARTESIAN_POINT('Ctrl Pts',(0.992206889613594,-1.76297069041634,
-7.48903838801854));
#363651=CARTESIAN_POINT('Ctrl Pts',(0.502190643379444,-1.95990154002328,
-7.51648926813145));
#363652=CARTESIAN_POINT('Ctrl Pts',(-0.0222096198383131,-2.0232383143754,
-7.54405136994835));
#363653=CARTESIAN_POINT('Ctrl Pts',(-0.545023222850085,-1.94828998299833,
-7.57157271170469));
#363654=CARTESIAN_POINT('Ctrl Pts',(-1.0307284358197,-1.74090605654878,
-7.59904290948243));
#363655=CARTESIAN_POINT('Ctrl Pts',(-1.44636321247892,-1.41496070139146,
-7.62658089390187));
#363656=CARTESIAN_POINT('Ctrl Pts',(-1.7630429012686,-0.992255621812916,
-7.65411407831587));
#363657=CARTESIAN_POINT('Ctrl Pts',(-1.95983623864864,-0.502172632985278,
-7.68158430816739));
#363658=CARTESIAN_POINT('Ctrl Pts',(-2.02326404614228,0.0222054813197516,
-7.70911956348259));
#363659=CARTESIAN_POINT('Ctrl Pts',(-1.94828990091774,0.545028935894718,
-7.73665436795491));
#363660=CARTESIAN_POINT('Ctrl Pts',(-1.74090287629493,1.03072354235614,
-7.76412460420479));
#363661=CARTESIAN_POINT('Ctrl Pts',(-1.41496257868532,1.44636639725859,
-7.79165822650409));
#363662=CARTESIAN_POINT('Ctrl Pts',(-0.992256976006747,1.76304240583952,
-7.81919574931953));
#363663=CARTESIAN_POINT('Ctrl Pts',(-0.502167983314945,1.95983220557862,
-7.84666606566923));
#363664=CARTESIAN_POINT('Ctrl Pts',(0.0222021542767409,2.02327125956959,
-7.87418752174917));
#363665=CARTESIAN_POINT('Ctrl Pts',(0.545036582780956,1.94830483935279,
-7.90174989061211));
#363666=CARTESIAN_POINT('Ctrl Pts',(1.03068639649234,1.74088018296961,-7.92919874059292));
#363667=CARTESIAN_POINT('Ctrl Pts',(1.41193217216583,1.44192597876132,-7.95443773023923));
#363668=CARTESIAN_POINT('Ctrl Pts',(1.68594383364152,1.10008635709056,-7.97735256352204));
#363669=CARTESIAN_POINT('Ctrl Pts',(1.86832284879594,0.749865410246654,
-7.99820416287286));
#363670=CARTESIAN_POINT('Ctrl Pts',(1.97885834740452,0.370827498858678,
-8.01808024799317));
#363671=CARTESIAN_POINT('Ctrl Pts',(2.00021510976845,0.108553308485772,
-8.03354455068052));
#363672=CARTESIAN_POINT('Ctrl Pts',(2.00021510976845,-0.0219451194485651,
-8.03925892415782));
#363673=CARTESIAN_POINT('Ctrl Pts',(2.80016361091613,-0.03493223178078,
-7.37981016006517));
#363674=CARTESIAN_POINT('Ctrl Pts',(2.80016361091613,-0.178346676400516,
-7.38609011080151));
#363675=CARTESIAN_POINT('Ctrl Pts',(2.75800714240104,-0.585623740854942,
-7.39993625174015));
#363676=CARTESIAN_POINT('Ctrl Pts',(2.59622001092688,-1.094203255455,-7.42050939398873));
#363677=CARTESIAN_POINT('Ctrl Pts',(2.33073889442298,-1.58539648585596,
-7.44121574714249));
#363678=CARTESIAN_POINT('Ctrl Pts',(1.93774673958377,-2.05527341692013,
-7.46406250879474));
#363679=CARTESIAN_POINT('Ctrl Pts',(1.3977924816811,-2.46335493607239,-7.4892382031805));
#363680=CARTESIAN_POINT('Ctrl Pts',(0.710887177607718,-2.74177962175189,
-7.51690579573811));
#363681=CARTESIAN_POINT('Ctrl Pts',(-0.0222315527777081,-2.83230238724503,
-7.54433060281804));
#363682=CARTESIAN_POINT('Ctrl Pts',(-0.753696284786715,-2.73017360349673,
-7.57179577476958));
#363683=CARTESIAN_POINT('Ctrl Pts',(-1.4359964022639,-2.44137112409355,
-7.59942818098223));
#363684=CARTESIAN_POINT('Ctrl Pts',(-2.01844596000972,-1.98707136838064,
-7.62687978029761));
#363685=CARTESIAN_POINT('Ctrl Pts',(-2.46348770759376,-1.39755415476222,
-7.65433629789662));
#363686=CARTESIAN_POINT('Ctrl Pts',(-2.74170364490091,-0.710913395495067,
-7.6819659616779));
#363687=CARTESIAN_POINT('Ctrl Pts',(-2.83233201369082,0.0221843029796173,
-7.70942122438771));
#363688=CARTESIAN_POINT('Ctrl Pts',(-2.73016814474818,0.753729685089645,
-7.73687603703565));
#363689=CARTESIAN_POINT('Ctrl Pts',(-2.44136831164089,1.43598613500131,
-7.76450570621253));
#363690=CARTESIAN_POINT('Ctrl Pts',(-1.98707527820992,2.01844704832099,
-7.79196266491878));
#363691=CARTESIAN_POINT('Ctrl Pts',(-1.39756088034447,2.46348708795637,
-7.8194137894634));
#363692=CARTESIAN_POINT('Ctrl Pts',(-0.710881081634362,2.74170412714945,
-7.84704636495045));
#363693=CARTESIAN_POINT('Ctrl Pts',(0.0221378788343896,2.83233850612441,
-7.87451146130275));
#363694=CARTESIAN_POINT('Ctrl Pts',(0.753693185451086,2.73018185071023,
-7.90193724347128));
#363695=CARTESIAN_POINT('Ctrl Pts',(1.43623604645724,2.44132953435746,-7.92960016599444));
#363696=CARTESIAN_POINT('Ctrl Pts',(1.96972754709332,2.02444453015913,-7.95479275010049));
#363697=CARTESIAN_POINT('Ctrl Pts',(2.35530318309127,1.54946734602988,-7.97759034640265));
#363698=CARTESIAN_POINT('Ctrl Pts',(2.61262613808022,1.05037578999858,-7.9984674292579));
#363699=CARTESIAN_POINT('Ctrl Pts',(2.76839001336968,0.552800283700582,
-8.01843767560678));
#363700=CARTESIAN_POINT('Ctrl Pts',(2.80021499480674,0.108538122595088,
-8.03388883389828));
#363701=CARTESIAN_POINT('Ctrl Pts',(2.80021499480674,-0.0219216792995908,
-8.0396015159865));
#363702=CARTESIAN_POINT('Ctrl Pts',(2.7998363224979,0.0349606549171637,
-8.01981010684661));
#363703=CARTESIAN_POINT('Ctrl Pts',(2.7998363224979,-0.108453789702572,
-8.02609005758295));
#363704=CARTESIAN_POINT('Ctrl Pts',(2.76770770092932,-0.554475300665122,
-8.04161041709402));
#363705=CARTESIAN_POINT('Ctrl Pts',(2.61230104920345,-1.04994348735895,
-8.06150470700589));
#363706=CARTESIAN_POINT('Ctrl Pts',(2.35499212095577,-1.5493099165356,-8.08239384111292));
#363707=CARTESIAN_POINT('Ctrl Pts',(1.96948131702204,-2.02412699417522,
-8.10518795929102));
#363708=CARTESIAN_POINT('Ctrl Pts',(1.43606137034988,-2.44099583455896,
-8.1303818337545));
#363709=CARTESIAN_POINT('Ctrl Pts',(0.753613249673498,-2.7298044063241,
-8.15804434422187));
#363710=CARTESIAN_POINT('Ctrl Pts',(0.0221607848766011,-2.83195604538419,
-8.18547015377513));
#363711=CARTESIAN_POINT('Ctrl Pts',(-0.710763089306898,-2.74133925166452,
-8.21293536328677));
#363712=CARTESIAN_POINT('Ctrl Pts',(-1.39735180486206,-2.46316525092768,
-8.24056787474674));
#363713=CARTESIAN_POINT('Ctrl Pts',(-1.9867882252217,-2.01819243450698,
-8.26801892009786));
#363714=CARTESIAN_POINT('Ctrl Pts',(-2.44102701245388,-1.43581160139486,
-8.2954760307671));
#363715=CARTESIAN_POINT('Ctrl Pts',(-2.72979268536681,-0.753649988228477,
-8.32310562488017));
#363716=CARTESIAN_POINT('Ctrl Pts',(-2.83194900848818,-0.022207241173352,
-8.35056035976573));
#363717=CARTESIAN_POINT('Ctrl Pts',(-2.74133888936392,0.710795480178799,
-8.37801577635552));
#363718=CARTESIAN_POINT('Ctrl Pts',(-2.4631658691281,1.3973450383548,-8.4056453623318));
#363719=CARTESIAN_POINT('Ctrl Pts',(-2.0181913618354,1.98678420052489,-8.43310180787527));
#363720=CARTESIAN_POINT('Ctrl Pts',(-1.43582178716812,2.44103031792683,
-8.4605535408052));
#363721=CARTESIAN_POINT('Ctrl Pts',(-0.753616702679641,2.7297964193171,
-8.48818595954062));
#363722=CARTESIAN_POINT('Ctrl Pts',(-0.0222544062348159,2.83192570994805,
-8.51565069030184));
#363723=CARTESIAN_POINT('Ctrl Pts',(0.710769507993571,2.74139122758401,
-8.54307702242869));
#363724=CARTESIAN_POINT('Ctrl Pts',(1.39758336815266,2.4631211079265,-8.5707395161615));
#363725=CARTESIAN_POINT('Ctrl Pts',(1.93746427579644,2.05471988808546,-8.59593214237152));
#363726=CARTESIAN_POINT('Ctrl Pts',(2.33041781164643,1.58599477455527,-8.61873057100975));
#363727=CARTESIAN_POINT('Ctrl Pts',(2.59583452983605,1.0910815303924,-8.63960593440206));
#363728=CARTESIAN_POINT('Ctrl Pts',(2.75797391874601,0.595981365328419,
-8.65957756239152));
#363729=CARTESIAN_POINT('Ctrl Pts',(2.79978489023148,0.152404921343189,
-8.67502839375386));
#363730=CARTESIAN_POINT('Ctrl Pts',(2.79978489023148,0.0219451194485099,
-8.68074107584208));
#363731=CARTESIAN_POINT('Ctrl Pts',(1.99983638908381,0.0349322317807904,
-8.0195498399348));
#363732=CARTESIAN_POINT('Ctrl Pts',(1.99983638908381,-0.10202602676277,
-8.02554708183654));
#363733=CARTESIAN_POINT('Ctrl Pts',(1.97826023278427,-0.374998458759011,
-8.04149750289518));
#363734=CARTESIAN_POINT('Ctrl Pts',(1.86797590755627,-0.748764460301907,
-8.06112897846829));
#363735=CARTESIAN_POINT('Ctrl Pts',(1.68561151450438,-1.10015061289253,
-8.08203775324541));
#363736=CARTESIAN_POINT('Ctrl Pts',(1.41165495945895,-1.44156834906321,
-8.10493617015518));
#363737=CARTESIAN_POINT('Ctrl Pts',(1.03047577828238,-1.74058787531436,
-8.13018098020224));
#363738=CARTESIAN_POINT('Ctrl Pts',(0.544916715445223,-1.94793268220013,
-8.15762809500727));
#363739=CARTESIAN_POINT('Ctrl Pts',(0.0221827178159963,-2.02289026809774,
-8.18519084627103));
#363740=CARTESIAN_POINT('Ctrl Pts',(-0.502090027370269,-1.95945608733342,
-8.21271232019691));
#363741=CARTESIAN_POINT('Ctrl Pts',(-0.992083838417867,-1.76270006106949,
-8.24018259789098));
#363742=CARTESIAN_POINT('Ctrl Pts',(-1.4147054776909,-1.44608180030657,
-8.26772003513789));
#363743=CARTESIAN_POINT('Ctrl Pts',(-1.74058220612872,-1.03051305966975,
-8.29525381080208));
#363744=CARTESIAN_POINT('Ctrl Pts',(-1.94792527911454,-0.54490922807225,
-8.32272397147271));
#363745=CARTESIAN_POINT('Ctrl Pts',(-2.02288104093964,-0.0221860622005593,
-8.3502586988329));
#363746=CARTESIAN_POINT('Ctrl Pts',(-1.95946064553349,0.502094730808056,
-8.37779410728247));
#363747=CARTESIAN_POINT('Ctrl Pts',(-1.76270043378214,0.992082445780963,
-8.40526426032094));
#363748=CARTESIAN_POINT('Ctrl Pts',(-1.4460786623108,1.41470354935293,-8.43279736946537));
#363749=CARTESIAN_POINT('Ctrl Pts',(-1.03051788283039,1.74058563617661,
-8.46033550064529));
#363750=CARTESIAN_POINT('Ctrl Pts',(-0.544903604360224,1.94792449639017,
-8.48780566031878));
#363751=CARTESIAN_POINT('Ctrl Pts',(-0.0221901307924648,2.02285846845712,
-8.51532675052651));
#363752=CARTESIAN_POINT('Ctrl Pts',(0.502112905323441,1.95951419733875,
-8.5428896703966));
#363753=CARTESIAN_POINT('Ctrl Pts',(0.992033718187761,1.76267182698944,
-8.57033808767502));
#363754=CARTESIAN_POINT('Ctrl Pts',(1.37966890086895,1.47220110119364,-8.59557713282226));
#363755=CARTESIAN_POINT('Ctrl Pts',(1.66105846219667,1.13661442398405,-8.61849276017575));
#363756=CARTESIAN_POINT('Ctrl Pts',(1.85153124055178,0.790568741290481,
-8.63934277351964));
#363757=CARTESIAN_POINT('Ctrl Pts',(1.96844225278085,0.414017589463527,
-8.65921974028535));
#363758=CARTESIAN_POINT('Ctrl Pts',(1.99978500519319,0.152400794214044,
-8.67468495623063));
#363759=CARTESIAN_POINT('Ctrl Pts',(1.99978500519318,0.0219216792995357,
-8.68039848401339));
#363760=CARTESIAN_POINT('Ctrl Pts',(1.19983645566973,0.0349038086444169,
-8.01928957302298));
#363761=CARTESIAN_POINT('Ctrl Pts',(1.19983645566973,-0.0955982638229683,
-8.02500410609012));
#363762=CARTESIAN_POINT('Ctrl Pts',(1.18881276463922,-0.1955216168529,-8.04138458869635));
#363763=CARTESIAN_POINT('Ctrl Pts',(1.12365076590908,-0.447585433244864,
-8.06075324993069));
#363764=CARTESIAN_POINT('Ctrl Pts',(1.016230908053,-0.650991309249464,-8.0816816653779));
#363765=CARTESIAN_POINT('Ctrl Pts',(0.853828601895857,-0.859009703951189,
-8.10468438101933));
#363766=CARTESIAN_POINT('Ctrl Pts',(0.624890186214873,-1.04017991606976,
-8.12998012664998));
#363767=CARTESIAN_POINT('Ctrl Pts',(0.336220181216949,-1.16606095807615,
-8.15721184579269));
#363768=CARTESIAN_POINT('Ctrl Pts',(0.0222046507553913,-1.21382449081129,
-8.18491153876691));
#363769=CARTESIAN_POINT('Ctrl Pts',(-0.29341696543364,-1.17757292300231,
-8.21248927710705));
#363770=CARTESIAN_POINT('Ctrl Pts',(-0.586815871973671,-1.0622348712113,
-8.23979732103521));
#363771=CARTESIAN_POINT('Ctrl Pts',(-0.842622730160096,-0.873971166106157,
-8.26742115017792));
#363772=CARTESIAN_POINT('Ctrl Pts',(-1.04013739980356,-0.625214517944632,
-8.29503159083705));
#363773=CARTESIAN_POINT('Ctrl Pts',(-1.16605787286226,-0.336168467916023,
-8.32234231806526));
#363774=CARTESIAN_POINT('Ctrl Pts',(-1.2138130733911,-0.0221648832277664,
-8.34995703790007));
#363775=CARTESIAN_POINT('Ctrl Pts',(-1.17758240170305,0.293393981437313,
-8.37757243820942));
#363776=CARTESIAN_POINT('Ctrl Pts',(-1.06223499843619,0.586819853207128,
-8.40488315831008));
#363777=CARTESIAN_POINT('Ctrl Pts',(-0.873965962786202,0.842622898180978,
-8.43249293105548));
#363778=CARTESIAN_POINT('Ctrl Pts',(-0.625213978492663,1.04014095442639,
-8.46011746048537));
#363779=CARTESIAN_POINT('Ctrl Pts',(-0.336190506040807,1.16605257346324,
-8.48742536109694));
#363780=CARTESIAN_POINT('Ctrl Pts',(-0.0221258553501136,1.21379122696619,
-8.51500281075118));
#363781=CARTESIAN_POINT('Ctrl Pts',(0.293456302653311,1.17763716709349,
-8.54270231836451));
#363782=CARTESIAN_POINT('Ctrl Pts',(0.586484068222858,1.06222254605237,
-8.56993665918854));
#363783=CARTESIAN_POINT('Ctrl Pts',(0.821873525941461,0.889682314301827,
-8.59522212327301));
#363784=CARTESIAN_POINT('Ctrl Pts',(0.991699112746911,0.687234073412837,
-8.61825494934175));
#363785=CARTESIAN_POINT('Ctrl Pts',(1.1072279512675,0.490055952188566,-8.63907961263722));
#363786=CARTESIAN_POINT('Ctrl Pts',(1.17891058681569,0.232053813598634,
-8.65886191817918));
#363787=CARTESIAN_POINT('Ctrl Pts',(1.19978512015489,0.152396667084899,
-8.6743415187074));
#363788=CARTESIAN_POINT('Ctrl Pts',(1.19978512015489,0.0218982391505614,
-8.6800558921847));
#363789=CARTESIAN_POINT('Ctrl Pts',(1.20016374408796,-0.0349890780535269,
-7.37928962624154));
#363790=CARTESIAN_POINT('Ctrl Pts',(1.20016374408796,-0.152578778368561,
-7.38443874163948));
#363791=CARTESIAN_POINT('Ctrl Pts',(1.17911220611093,-0.232722898983027,
-7.39997547020929));
#363792=CARTESIAN_POINT('Ctrl Pts',(1.1075697276325,-0.490223236218595,
-7.41968691295851));
#363793=CARTESIAN_POINT('Ctrl Pts',(0.99197768152021,-0.687507626341548,
-7.44052238955959));
#363794=CARTESIAN_POINT('Ctrl Pts',(0.822094024457586,-0.889997593033309,
-7.46355198851942));
#363795=CARTESIAN_POINT('Ctrl Pts',(0.586621297546092,-1.06258644476029,
-7.48883857285657));
#363796=CARTESIAN_POINT('Ctrl Pts',(0.293494109151169,-1.17802345829468,
-7.51607274052479));
#363797=CARTESIAN_POINT('Ctrl Pts',(-0.022187686898918,-1.21417424150576,
-7.54377213707865));
#363798=CARTESIAN_POINT('Ctrl Pts',(-0.336350160913456,-1.16640636249992,
-7.5713496486398));
#363799=CARTESIAN_POINT('Ctrl Pts',(-0.625460469375504,-1.04044098900401,
-7.59865763798262));
#363800=CARTESIAN_POINT('Ctrl Pts',(-0.874280464948115,-0.842850034402287,
-7.62628200750612));
#363801=CARTESIAN_POINT('Ctrl Pts',(-1.06259809494344,-0.586957088863615,
-7.65389185873512));
#363802=CARTESIAN_POINT('Ctrl Pts',(-1.17796883239637,-0.293431870475487,
-7.68120265465688));
#363803=CARTESIAN_POINT('Ctrl Pts',(-1.21419607859374,0.0222266596598858,
-7.70881790257747));
#363804=CARTESIAN_POINT('Ctrl Pts',(-1.16641165708731,0.33632818669979,
-7.73643269887416));
#363805=CARTESIAN_POINT('Ctrl Pts',(-1.04043744094898,0.625460949710965,
-7.76374350219705));
#363806=CARTESIAN_POINT('Ctrl Pts',(-0.842849879160721,0.874285746196179,
-7.7913537880894));
#363807=CARTESIAN_POINT('Ctrl Pts',(-0.58695307166902,1.06259772372267,
-7.81897770917568));
#363808=CARTESIAN_POINT('Ctrl Pts',(-0.293454884995528,1.17796028400778,
-7.846285766388));
#363809=CARTESIAN_POINT('Ctrl Pts',(0.0222664297190919,1.21420401301477,
-7.87386358219558));
#363810=CARTESIAN_POINT('Ctrl Pts',(0.336379980110826,1.16642782799535,
-7.90156253775294));
#363811=CARTESIAN_POINT('Ctrl Pts',(0.625136746527436,1.04043083158176,
-7.9287973151914));
#363812=CARTESIAN_POINT('Ctrl Pts',(0.854136797238339,0.859407427363523,
-7.95408271037797));
#363813=CARTESIAN_POINT('Ctrl Pts',(1.01658448419176,0.650705368151239,
-7.97711478064143));
#363814=CARTESIAN_POINT('Ctrl Pts',(1.12401955951167,0.449355030494726,
-7.99794089648783));
#363815=CARTESIAN_POINT('Ctrl Pts',(1.18932668143936,0.188854714016773,
-8.01772282037956));
#363816=CARTESIAN_POINT('Ctrl Pts',(1.20021522473016,0.108568494376457,
-8.03320026746274));
#363817=CARTESIAN_POINT('Ctrl Pts',(1.20021522473015,-0.0219685595975393,
-8.03891633232913));
#363818=CARTESIAN_POINT('Ctrl Pts',(2.00016367750204,-0.0349606549171534,
-7.37954989315335));
#363819=CARTESIAN_POINT('Ctrl Pts',(2.00016367750204,-0.165462727384539,
-7.38526442622049));
#363820=CARTESIAN_POINT('Ctrl Pts',(1.96855967425598,-0.409173319918984,
-7.39995586097472));
#363821=CARTESIAN_POINT('Ctrl Pts',(1.85189486927969,-0.792213245836797,
-7.42009815347362));
#363822=CARTESIAN_POINT('Ctrl Pts',(1.6613582879716,-1.13645205609876,-7.44086906835104));
#363823=CARTESIAN_POINT('Ctrl Pts',(1.37992038202068,-1.47263550497672,
-7.46380724865708));
#363824=CARTESIAN_POINT('Ctrl Pts',(0.992206889613594,-1.76297069041634,
-7.48903838801854));
#363825=CARTESIAN_POINT('Ctrl Pts',(0.502190643379444,-1.95990154002328,
-7.51648926813145));
#363826=CARTESIAN_POINT('Ctrl Pts',(-0.0222096198383131,-2.0232383143754,
-7.54405136994835));
#363827=CARTESIAN_POINT('Ctrl Pts',(-0.545023222850085,-1.94828998299833,
-7.57157271170469));
#363828=CARTESIAN_POINT('Ctrl Pts',(-1.0307284358197,-1.74090605654878,
-7.59904290948243));
#363829=CARTESIAN_POINT('Ctrl Pts',(-1.44636321247892,-1.41496070139146,
-7.62658089390187));
#363830=CARTESIAN_POINT('Ctrl Pts',(-1.7630429012686,-0.992255621812916,
-7.65411407831587));
#363831=CARTESIAN_POINT('Ctrl Pts',(-1.95983623864864,-0.502172632985278,
-7.68158430816739));
#363832=CARTESIAN_POINT('Ctrl Pts',(-2.02326404614228,0.0222054813197516,
-7.70911956348259));
#363833=CARTESIAN_POINT('Ctrl Pts',(-1.94828990091774,0.545028935894718,
-7.73665436795491));
#363834=CARTESIAN_POINT('Ctrl Pts',(-1.74090287629493,1.03072354235614,
-7.76412460420479));
#363835=CARTESIAN_POINT('Ctrl Pts',(-1.41496257868532,1.44636639725859,
-7.79165822650409));
#363836=CARTESIAN_POINT('Ctrl Pts',(-0.992256976006747,1.76304240583952,
-7.81919574931953));
#363837=CARTESIAN_POINT('Ctrl Pts',(-0.502167983314945,1.95983220557862,
-7.84666606566923));
#363838=CARTESIAN_POINT('Ctrl Pts',(0.0222021542767409,2.02327125956959,
-7.87418752174917));
#363839=CARTESIAN_POINT('Ctrl Pts',(0.545036582780956,1.94830483935279,
-7.90174989061211));
#363840=CARTESIAN_POINT('Ctrl Pts',(1.03068639649234,1.74088018296961,-7.92919874059292));
#363841=CARTESIAN_POINT('Ctrl Pts',(1.41193217216583,1.44192597876132,-7.95443773023923));
#363842=CARTESIAN_POINT('Ctrl Pts',(1.68594383364152,1.10008635709056,-7.97735256352204));
#363843=CARTESIAN_POINT('Ctrl Pts',(1.86832284879594,0.749865410246654,
-7.99820416287286));
#363844=CARTESIAN_POINT('Ctrl Pts',(1.97885834740452,0.370827498858678,
-8.01808024799317));
#363845=CARTESIAN_POINT('Ctrl Pts',(2.00021510976845,0.108553308485772,
-8.03354455068052));
#363846=CARTESIAN_POINT('Ctrl Pts',(2.00021510976845,-0.0219451194485651,
-8.03925892415782));
#363847=CARTESIAN_POINT('',(1.99983638908381,0.0349322317806574,-8.0195498399348));
#363848=CARTESIAN_POINT('',(1.6000000331116,-1.41261775450829E-5,-7.6995506484554));
#363849=CARTESIAN_POINT('Origin',(2.00000003329293,-1.42115683144772E-5,
-7.69954986654408));
#363850=CARTESIAN_POINT('',(1.99978500519318,0.0219216792995357,-8.68039848401339));
#363851=CARTESIAN_POINT('Ctrl Pts',(1.99983638908381,0.0349322317806574,
-8.0195498399348));
#363852=CARTESIAN_POINT('Ctrl Pts',(1.99983638908381,-0.10202602676277,
-8.02554708183654));
#363853=CARTESIAN_POINT('Ctrl Pts',(1.97826023278427,-0.374998458759011,
-8.04149750289518));
#363854=CARTESIAN_POINT('Ctrl Pts',(1.86797590755627,-0.748764460301907,
-8.06112897846829));
#363855=CARTESIAN_POINT('Ctrl Pts',(1.68561151450438,-1.10015061289253,
-8.08203775324541));
#363856=CARTESIAN_POINT('Ctrl Pts',(1.41165495945895,-1.44156834906321,
-8.10493617015518));
#363857=CARTESIAN_POINT('Ctrl Pts',(1.03047577828238,-1.74058787531436,
-8.13018098020224));
#363858=CARTESIAN_POINT('Ctrl Pts',(0.544916715445223,-1.94793268220013,
-8.15762809500727));
#363859=CARTESIAN_POINT('Ctrl Pts',(0.0221827178159963,-2.02289026809774,
-8.18519084627103));
#363860=CARTESIAN_POINT('Ctrl Pts',(-0.502090027370269,-1.95945608733342,
-8.21271232019691));
#363861=CARTESIAN_POINT('Ctrl Pts',(-0.992083838417867,-1.76270006106949,
-8.24018259789098));
#363862=CARTESIAN_POINT('Ctrl Pts',(-1.4147054776909,-1.44608180030657,
-8.26772003513789));
#363863=CARTESIAN_POINT('Ctrl Pts',(-1.74058220612872,-1.03051305966975,
-8.29525381080208));
#363864=CARTESIAN_POINT('Ctrl Pts',(-1.94792527911454,-0.54490922807225,
-8.32272397147271));
#363865=CARTESIAN_POINT('Ctrl Pts',(-2.02288104093964,-0.0221860622005593,
-8.3502586988329));
#363866=CARTESIAN_POINT('Ctrl Pts',(-1.95946064553349,0.502094730808056,
-8.37779410728247));
#363867=CARTESIAN_POINT('Ctrl Pts',(-1.76270043378214,0.992082445780963,
-8.40526426032094));
#363868=CARTESIAN_POINT('Ctrl Pts',(-1.4460786623108,1.41470354935293,-8.43279736946537));
#363869=CARTESIAN_POINT('Ctrl Pts',(-1.03051788283039,1.74058563617661,
-8.46033550064529));
#363870=CARTESIAN_POINT('Ctrl Pts',(-0.544903604360224,1.94792449639017,
-8.48780566031878));
#363871=CARTESIAN_POINT('Ctrl Pts',(-0.0221901307924648,2.02285846845712,
-8.51532675052651));
#363872=CARTESIAN_POINT('Ctrl Pts',(0.502112905323441,1.95951419733875,
-8.5428896703966));
#363873=CARTESIAN_POINT('Ctrl Pts',(0.992033718187761,1.76267182698944,
-8.57033808767502));
#363874=CARTESIAN_POINT('Ctrl Pts',(1.37966890086895,1.47220110119364,-8.59557713282226));
#363875=CARTESIAN_POINT('Ctrl Pts',(1.66105846219667,1.13661442398405,-8.61849276017575));
#363876=CARTESIAN_POINT('Ctrl Pts',(1.85153124055178,0.790568741290481,
-8.63934277351964));
#363877=CARTESIAN_POINT('Ctrl Pts',(1.96844225278085,0.414017589463527,
-8.65921974028535));
#363878=CARTESIAN_POINT('Ctrl Pts',(1.99978500519319,0.152400794214044,
-8.67468495623063));
#363879=CARTESIAN_POINT('Ctrl Pts',(1.99978500519318,0.0219216792995357,
-8.68039848401339));
#363880=CARTESIAN_POINT('',(2.00021510976845,-0.0219451194485651,-8.03925892415782));
#363881=CARTESIAN_POINT('Origin',(2.00000005748082,-1.17200745146546E-5,
-8.35982870408561));
#363882=CARTESIAN_POINT('',(2.00016367750204,-0.0349606549172864,-7.37954989315336));
#363883=CARTESIAN_POINT('Ctrl Pts',(2.00016367750204,-0.0349606549172864,
-7.37954989315336));
#363884=CARTESIAN_POINT('Ctrl Pts',(2.00016367750204,-0.165462727384539,
-7.38526442622049));
#363885=CARTESIAN_POINT('Ctrl Pts',(1.96855967425598,-0.409173319918984,
-7.39995586097472));
#363886=CARTESIAN_POINT('Ctrl Pts',(1.85189486927969,-0.792213245836797,
-7.42009815347362));
#363887=CARTESIAN_POINT('Ctrl Pts',(1.6613582879716,-1.13645205609876,-7.44086906835104));
#363888=CARTESIAN_POINT('Ctrl Pts',(1.37992038202068,-1.47263550497672,
-7.46380724865708));
#363889=CARTESIAN_POINT('Ctrl Pts',(0.992206889613594,-1.76297069041634,
-7.48903838801854));
#363890=CARTESIAN_POINT('Ctrl Pts',(0.502190643379444,-1.95990154002328,
-7.51648926813145));
#363891=CARTESIAN_POINT('Ctrl Pts',(-0.0222096198383131,-2.0232383143754,
-7.54405136994835));
#363892=CARTESIAN_POINT('Ctrl Pts',(-0.545023222850085,-1.94828998299833,
-7.57157271170469));
#363893=CARTESIAN_POINT('Ctrl Pts',(-1.0307284358197,-1.74090605654878,
-7.59904290948243));
#363894=CARTESIAN_POINT('Ctrl Pts',(-1.44636321247892,-1.41496070139146,
-7.62658089390187));
#363895=CARTESIAN_POINT('Ctrl Pts',(-1.7630429012686,-0.992255621812916,
-7.65411407831587));
#363896=CARTESIAN_POINT('Ctrl Pts',(-1.95983623864864,-0.502172632985277,
-7.68158430816739));
#363897=CARTESIAN_POINT('Ctrl Pts',(-2.02326404614228,0.0222054813197516,
-7.70911956348259));
#363898=CARTESIAN_POINT('Ctrl Pts',(-1.94828990091774,0.545028935894718,
-7.73665436795491));
#363899=CARTESIAN_POINT('Ctrl Pts',(-1.74090287629493,1.03072354235614,
-7.76412460420479));
#363900=CARTESIAN_POINT('Ctrl Pts',(-1.41496257868532,1.44636639725859,
-7.79165822650409));
#363901=CARTESIAN_POINT('Ctrl Pts',(-0.992256976006747,1.76304240583952,
-7.81919574931953));
#363902=CARTESIAN_POINT('Ctrl Pts',(-0.502167983314945,1.95983220557862,
-7.84666606566923));
#363903=CARTESIAN_POINT('Ctrl Pts',(0.0222021542767409,2.02327125956959,
-7.87418752174917));
#363904=CARTESIAN_POINT('Ctrl Pts',(0.545036582780956,1.94830483935279,
-7.90174989061211));
#363905=CARTESIAN_POINT('Ctrl Pts',(1.03068639649234,1.74088018296961,-7.92919874059292));
#363906=CARTESIAN_POINT('Ctrl Pts',(1.41193217216583,1.44192597876132,-7.95443773023923));
#363907=CARTESIAN_POINT('Ctrl Pts',(1.68594383364152,1.10008635709056,-7.97735256352204));
#363908=CARTESIAN_POINT('Ctrl Pts',(1.86832284879594,0.749865410246654,
-7.99820416287286));
#363909=CARTESIAN_POINT('Ctrl Pts',(1.97885834740452,0.370827498858678,
-8.01808024799317));
#363910=CARTESIAN_POINT('Ctrl Pts',(2.00021510976845,0.108553308485772,
-8.03354455068052));
#363911=CARTESIAN_POINT('Ctrl Pts',(2.00021510976845,-0.0219451194485651,
-8.03925892415782));
#363912=CARTESIAN_POINT('Origin',(2.00000003329293,-1.42115683144772E-5,
-7.69954986654408));
#363913=CARTESIAN_POINT('Ctrl Pts',(2.00005141137773,-0.0349509159166537,
-1.58027907189674));
#363914=CARTESIAN_POINT('Ctrl Pts',(2.00005141137773,-0.209477500702,-1.59705901785001));
#363915=CARTESIAN_POINT('Ctrl Pts',(1.93937485936534,-0.574981221086946,
-1.64398167301615));
#363916=CARTESIAN_POINT('Ctrl Pts',(1.72866575619624,-1.05218683017129,
-1.70157781695483));
#363917=CARTESIAN_POINT('Ctrl Pts',(1.39603065320521,-1.46514475575449,
-1.76296158741006));
#363918=CARTESIAN_POINT('Ctrl Pts',(0.969522180315677,-1.77589106055163,
-1.82311912419573));
#363919=CARTESIAN_POINT('Ctrl Pts',(0.476783238604109,-1.96670288995313,
-1.88346520364747));
#363920=CARTESIAN_POINT('Ctrl Pts',(-0.0484603850821368,-2.02312932285366,
-1.94396055370022));
#363921=CARTESIAN_POINT('Ctrl Pts',(-0.570338856925993,-1.94138942628423,
-2.00439291407465));
#363922=CARTESIAN_POINT('Ctrl Pts',(-1.05344948325284,-1.72773686772633,
-2.06470891120488));
#363923=CARTESIAN_POINT('Ctrl Pts',(-1.46487312544728,-1.39632835696345,
-2.1251726344757));
#363924=CARTESIAN_POINT('Ctrl Pts',(-1.77606001340043,-0.969474639293403,
-2.18562457894241));
#363925=CARTESIAN_POINT('Ctrl Pts',(-1.9665886161183,-0.476795144252666,
-2.2459421237894));
#363926=CARTESIAN_POINT('Ctrl Pts',(-2.0231790616074,0.0484698229690482,
-2.30639998925771));
#363927=CARTESIAN_POINT('Ctrl Pts',(-1.94138573006516,0.570342005097921,
-2.36685494461854));
#363928=CARTESIAN_POINT('Ctrl Pts',(-1.72773301625381,1.05344259449438,
-2.42717237256682));
#363929=CARTESIAN_POINT('Ctrl Pts',(-1.39633042998923,1.46487729238585,
-2.48762977035772));
#363930=CARTESIAN_POINT('Ctrl Pts',(-0.969474291036093,1.77605966206198,
-2.54808497616048));
#363931=CARTESIAN_POINT('Ctrl Pts',(-0.476795343347378,1.96658811640277,
-2.6084023881129));
#363932=CARTESIAN_POINT('Ctrl Pts',(0.0484699602192744,2.02317939996145,
-2.66885975673847));
#363933=CARTESIAN_POINT('Ctrl Pts',(0.570341982836039,1.94138567238666,
-2.72931497821885));
#363934=CARTESIAN_POINT('Ctrl Pts',(1.05344257210098,1.72773301387229,-2.78963238875962));
#363935=CARTESIAN_POINT('Ctrl Pts',(1.46487731147791,1.39633043581364,-2.85008975616076));
#363936=CARTESIAN_POINT('Ctrl Pts',(1.7760596572503,0.96947429019414,-2.91054497830833));
#363937=CARTESIAN_POINT('Ctrl Pts',(1.96658811657123,0.47679534386094,-2.97086238877306));
#363938=CARTESIAN_POINT('Ctrl Pts',(2.02317940049204,-0.0484699606166185,
-3.03131975614836));
#363939=CARTESIAN_POINT('Ctrl Pts',(1.94138567221384,-0.570341982644115,
-3.09177497831011));
#363940=CARTESIAN_POINT('Ctrl Pts',(1.72773301391076,-1.05344257214956,
-3.15209238877301));
#363941=CARTESIAN_POINT('Ctrl Pts',(1.39633043580907,-1.46487731147983,
-3.21254975614839));
#363942=CARTESIAN_POINT('Ctrl Pts',(0.969474290197969,-1.77605965724421,
-3.27300497831004));
#363943=CARTESIAN_POINT('Ctrl Pts',(0.476795343858464,-1.96658811657341,
-3.33332238877311));
#363944=CARTESIAN_POINT('Ctrl Pts',(-0.0484699606159255,-2.0231794004916,
-3.39377975614832));
#363945=CARTESIAN_POINT('Ctrl Pts',(-0.570341982644268,-1.94138567221424,
-3.45423497831005));
#363946=CARTESIAN_POINT('Ctrl Pts',(-1.05344257214943,-1.72773301391041,
-3.51455238877311));
#363947=CARTESIAN_POINT('Ctrl Pts',(-1.46487731147993,-1.39633043580919,
-3.57500975614831));
#363948=CARTESIAN_POINT('Ctrl Pts',(-1.77605965724425,-0.969474290197954,
-3.63546497831004));
#363949=CARTESIAN_POINT('Ctrl Pts',(-1.96658811657337,-0.476795343858458,
-3.69578238877312));
#363950=CARTESIAN_POINT('Ctrl Pts',(-2.02317940049162,0.0484699606159343,
-3.75623975614831));
#363951=CARTESIAN_POINT('Ctrl Pts',(-1.94138567221425,0.570341982644281,
-3.81669497831005));
#363952=CARTESIAN_POINT('Ctrl Pts',(-1.7277330139104,1.05344257214943,-3.87701238877311));
#363953=CARTESIAN_POINT('Ctrl Pts',(-1.39633043580919,1.46487731147993,
-3.93746975614831));
#363954=CARTESIAN_POINT('Ctrl Pts',(-0.969474290197942,1.77605965724426,
-3.99792497831004));
#363955=CARTESIAN_POINT('Ctrl Pts',(-0.476795343858452,1.96658811657335,
-4.05824238877313));
#363956=CARTESIAN_POINT('Ctrl Pts',(0.0484699606159434,2.02317940049163,
-4.11869975614831));
#363957=CARTESIAN_POINT('Ctrl Pts',(0.570341982644284,1.94138567221424,
-4.17915497831005));
#363958=CARTESIAN_POINT('Ctrl Pts',(1.05344257214943,1.72773301391039,-4.23947238877311));
#363959=CARTESIAN_POINT('Ctrl Pts',(1.46487731147993,1.39633043580918,-4.29992975614832));
#363960=CARTESIAN_POINT('Ctrl Pts',(1.77605965724427,0.969474290197945,
-4.36038497831003));
#363961=CARTESIAN_POINT('Ctrl Pts',(1.96658811657337,0.476795343858441,
-4.42070238877312));
#363962=CARTESIAN_POINT('Ctrl Pts',(2.02317940049162,-0.0484699606159445,
-4.48115975614831));
#363963=CARTESIAN_POINT('Ctrl Pts',(1.94138567221424,-0.570341982644292,
-4.54161497831005));
#363964=CARTESIAN_POINT('Ctrl Pts',(1.72773301391038,-1.05344257214943,
-4.60193238877312));
#363965=CARTESIAN_POINT('Ctrl Pts',(1.39633043580918,-1.46487731147994,
-4.66238975614831));
#363966=CARTESIAN_POINT('Ctrl Pts',(0.969474290197935,-1.77605965724426,
-4.72284497831004));
#363967=CARTESIAN_POINT('Ctrl Pts',(0.476795343858439,-1.96658811657337,
-4.78316238877312));
#363968=CARTESIAN_POINT('Ctrl Pts',(-0.0484699606159579,-2.02317940049164,
-4.8436197561483));
#363969=CARTESIAN_POINT('Ctrl Pts',(-0.570341982644288,-1.94138567221422,
-4.90407497831006));
#363970=CARTESIAN_POINT('Ctrl Pts',(-1.05344257214943,-1.72773301391037,
-4.96439238877312));
#363971=CARTESIAN_POINT('Ctrl Pts',(-1.46487731147995,-1.39633043580918,
-5.02484975614831));
#363972=CARTESIAN_POINT('Ctrl Pts',(-1.77605965724426,-0.969474290197928,
-5.08530497831004));
#363973=CARTESIAN_POINT('Ctrl Pts',(-1.96658811657335,-0.476795343858433,
-5.14562238877313));
#363974=CARTESIAN_POINT('Ctrl Pts',(-2.02317940049163,0.0484699606159606,
-5.2060797561483));
#363975=CARTESIAN_POINT('Ctrl Pts',(-1.94138567221425,0.570341982644311,
-5.26653497831003));
#363976=CARTESIAN_POINT('Ctrl Pts',(-1.72773301391036,1.05344257214944,
-5.32685238877313));
#363977=CARTESIAN_POINT('Ctrl Pts',(-1.39633043580918,1.46487731147996,
-5.3873097561483));
#363978=CARTESIAN_POINT('Ctrl Pts',(-0.969474290197916,1.77605965724424,
-5.44776497831006));
#363979=CARTESIAN_POINT('Ctrl Pts',(-0.476795343858422,1.96658811657339,
-5.5080823887731));
#363980=CARTESIAN_POINT('Ctrl Pts',(0.0484699606159706,2.02317940049163,
-5.56853975614829));
#363981=CARTESIAN_POINT('Ctrl Pts',(0.570341982644291,1.94138567221422,
-5.62899497831007));
#363982=CARTESIAN_POINT('Ctrl Pts',(1.05344257214944,1.72773301391032,-5.68931238877313));
#363983=CARTESIAN_POINT('Ctrl Pts',(1.46487731147996,1.3963304358092,-5.74976975614823));
#363984=CARTESIAN_POINT('Ctrl Pts',(1.77605965724441,0.969474290197947,
-5.81022497831013));
#363985=CARTESIAN_POINT('Ctrl Pts',(1.96658811657315,0.476795343858267,
-5.87054238877304));
#363986=CARTESIAN_POINT('Ctrl Pts',(2.02317940049197,-0.0484699606151168,
-5.93099975614826));
#363987=CARTESIAN_POINT('Ctrl Pts',(1.94138567221262,-0.570341982647331,
-5.99145497831012));
#363988=CARTESIAN_POINT('Ctrl Pts',(1.72773301391079,-1.05344257214282,
-6.05177238877488));
#363989=CARTESIAN_POINT('Ctrl Pts',(1.39633043583791,-1.46487731150212,
-6.1122297561358));
#363990=CARTESIAN_POINT('Ctrl Pts',(0.969474290103704,-1.77605965719443,
-6.17268497832268));
#363991=CARTESIAN_POINT('Ctrl Pts',(0.476795344014053,-1.96658811647506,
-6.23300238886911));
#363992=CARTESIAN_POINT('Ctrl Pts',(-0.0484699607888847,-2.02317940162764,
-6.293459755551));
#363993=CARTESIAN_POINT('Ctrl Pts',(-0.570341982515374,-1.94138566986718,
-6.35391497894857));
#363994=CARTESIAN_POINT('Ctrl Pts',(-1.0534425689941,-1.72773301427299,
-6.41423239105532));
#363995=CARTESIAN_POINT('Ctrl Pts',(-1.46487733129139,-1.39633044764682,
-6.47468974174144));
#363996=CARTESIAN_POINT('Ctrl Pts',(-1.77605962440754,-0.969474272408487,
-6.53514499410053));
#363997=CARTESIAN_POINT('Ctrl Pts',(-1.96658808441403,-0.4767953693466,
-6.59546242507117));
#363998=CARTESIAN_POINT('Ctrl Pts',(-2.02317971788315,0.0484700612956726,
-6.65591951867769));
#363999=CARTESIAN_POINT('Ctrl Pts',(-1.94138529374751,0.57034175258804,
-6.71637524065362));
#364000=CARTESIAN_POINT('Ctrl Pts',(-1.7277327906675,1.05344225923825,-6.77669281345839));
#364001=CARTESIAN_POINT('Ctrl Pts',(-1.39633190064527,1.46488023063332,
-6.83714685373563));
#364002=CARTESIAN_POINT('Ctrl Pts',(-0.969474795144666,1.77605674551469,
-6.89760831895014));
#364003=CARTESIAN_POINT('Ctrl Pts',(-0.476792483974202,1.96658170561334,
-6.95792512927773));
#364004=CARTESIAN_POINT('Ctrl Pts',(0.0484734593030573,2.0232081210323,
-7.01835708981697));
#364005=CARTESIAN_POINT('Ctrl Pts',(0.570336624689882,1.94136175768686,
-7.07885725203471));
#364006=CARTESIAN_POINT('Ctrl Pts',(1.05340619968671,1.72778052727257,-7.13918044053492));
#364007=CARTESIAN_POINT('Ctrl Pts',(1.46503146071072,1.39600002911185,-7.19942807213429));
#364008=CARTESIAN_POINT('Ctrl Pts',(1.77572739170825,0.970967789756964,
-7.26046972816476));
#364009=CARTESIAN_POINT('Ctrl Pts',(1.9679960876878,0.471734127632586,-7.31921124624962));
#364010=CARTESIAN_POINT('Ctrl Pts',(2.00016367750205,0.139563645186354,
-7.36277016686196));
#364011=CARTESIAN_POINT('Ctrl Pts',(2.00016367750204,-0.0349606549172864,
-7.37954989315336));
#364012=CARTESIAN_POINT('Ctrl Pts',(1.20005141796495,-0.0349598558146385,
-1.58019721042982));
#364013=CARTESIAN_POINT('Ctrl Pts',(1.20005141796495,-0.196639509400045,
-1.59574198174499));
#364014=CARTESIAN_POINT('Ctrl Pts',(1.15732797686238,-0.340816716447164,
-1.6447382432052));
#364015=CARTESIAN_POINT('Ctrl Pts',(1.02794595474197,-0.654182454634222,
-1.70085757593186));
#364016=CARTESIAN_POINT('Ctrl Pts',(0.824371570064879,-0.890750973398493,
-1.76298366242172));
#364017=CARTESIAN_POINT('Ctrl Pts',(0.563969291479731,-1.07614468532721,
-1.82314153495176));
#364018=CARTESIAN_POINT('Ctrl Pts',(0.268053015090469,-1.18466145511491,
-1.88305373693166));
#364019=CARTESIAN_POINT('Ctrl Pts',(-0.0484395870237313,-1.21410753423567,
-1.9438363016732));
#364020=CARTESIAN_POINT('Ctrl Pts',(-0.361651032204537,-1.15949959431507,
-2.00439370017114));
#364021=CARTESIAN_POINT('Ctrl Pts',(-0.648204859882796,-1.02726348852071,
-2.06435695179187));
#364022=CARTESIAN_POINT('Ctrl Pts',(-0.892791267502041,-0.824210832808723,
-2.12500826054469));
#364023=CARTESIAN_POINT('Ctrl Pts',(-1.07560894612736,-0.564190577762509,
-2.18562659547641));
#364024=CARTESIAN_POINT('Ctrl Pts',(-1.1847293912525,-0.268030428045687,
-2.24559800960236));
#364025=CARTESIAN_POINT('Ctrl Pts',(-1.21410751416084,0.0484963826130714,
-2.30623010797513));
#364026=CARTESIAN_POINT('Ctrl Pts',(-1.1595132046369,0.36162639690026,-2.36685750692005));
#364027=CARTESIAN_POINT('Ctrl Pts',(-1.02725604518277,0.648203827608334,
-2.42682890216184));
#364028=CARTESIAN_POINT('Ctrl Pts',(-0.824211659423609,0.892796064601774,
-2.48745940373019));
#364029=CARTESIAN_POINT('Ctrl Pts',(-0.564191142051916,1.07560808882016,
-2.54808760329284));
#364030=CARTESIAN_POINT('Ctrl Pts',(-0.268030403610479,1.18472901687534,
-2.60805895542665));
#364031=CARTESIAN_POINT('Ctrl Pts',(0.0484964956129267,1.21410782343574,
-2.66868935921047));
#364032=CARTESIAN_POINT('Ctrl Pts',(0.361626396132377,1.15951315047799,
-2.72931761037603));
#364033=CARTESIAN_POINT('Ctrl Pts',(0.648203803824844,1.0272560382112,-2.78928895746987));
#364034=CARTESIAN_POINT('Ctrl Pts',(0.892796076188025,0.824211675103123,
-2.84991935728737));
#364035=CARTESIAN_POINT('Ctrl Pts',(1.07560808862158,0.56419113400383,-2.91054761072926));
#364036=CARTESIAN_POINT('Ctrl Pts',(1.18472901588199,0.26803040550146,-2.97051895749492));
#364037=CARTESIAN_POINT('Ctrl Pts',(1.21410782431058,-0.0484964950668307,
-3.03114935724649));
#364038=CARTESIAN_POINT('Ctrl Pts',(1.15951315008857,-0.361626396645578,
-3.09177761073831));
#364039=CARTESIAN_POINT('Ctrl Pts',(1.02725603829716,-0.6482038036989,-3.15174895749339));
#364040=CARTESIAN_POINT('Ctrl Pts',(0.824211675135244,-0.892796076188428,
-3.21237935724692));
#364041=CARTESIAN_POINT('Ctrl Pts',(0.564191133978922,-1.07560808862653,
-3.27300761073802));
#364042=CARTESIAN_POINT('Ctrl Pts',(0.268030405508416,-1.18472901588096,
-3.33297895749366));
#364043=CARTESIAN_POINT('Ctrl Pts',(-0.0484964950686988,-1.21410782431092,
-3.39360935724675));
#364044=CARTESIAN_POINT('Ctrl Pts',(-0.361626396644909,-1.15951315008879,
-3.45423761073805));
#364045=CARTESIAN_POINT('Ctrl Pts',(-0.648203803698724,-1.02725603829705,
-3.51420895749367));
#364046=CARTESIAN_POINT('Ctrl Pts',(-0.89279607618879,-0.824211675135025,
-3.57483935724674));
#364047=CARTESIAN_POINT('Ctrl Pts',(-1.07560808862643,-0.564191133979103,
-3.63546761073801));
#364048=CARTESIAN_POINT('Ctrl Pts',(-1.18472901588094,-0.26803040550839,
-3.6954389574937));
#364049=CARTESIAN_POINT('Ctrl Pts',(-1.21410782431094,0.0484964950687397,
-3.75606935724672));
#364050=CARTESIAN_POINT('Ctrl Pts',(-1.1595131500888,0.361626396644898,
-3.81669761073803));
#364051=CARTESIAN_POINT('Ctrl Pts',(-1.02725603829704,0.648203803698727,
-3.87666895749368));
#364052=CARTESIAN_POINT('Ctrl Pts',(-0.824211675135021,0.892796076188792,
-3.93729935724673));
#364053=CARTESIAN_POINT('Ctrl Pts',(-0.564191133979095,1.07560808862643,
-3.99792761073801));
#364054=CARTESIAN_POINT('Ctrl Pts',(-0.268030405508389,1.18472901588092,
-4.05789895749373));
#364055=CARTESIAN_POINT('Ctrl Pts',(0.0484964950687464,1.21410782431094,
-4.11852935724671));
#364056=CARTESIAN_POINT('Ctrl Pts',(0.3616263966449,1.15951315008879,-4.17915761073805));
#364057=CARTESIAN_POINT('Ctrl Pts',(0.648203803698728,1.02725603829704,
-4.23912895749368));
#364058=CARTESIAN_POINT('Ctrl Pts',(0.892796076188791,0.824211675135014,
-4.29975935724674));
#364059=CARTESIAN_POINT('Ctrl Pts',(1.07560808862644,0.564191133979099,
-4.36038761073799));
#364060=CARTESIAN_POINT('Ctrl Pts',(1.18472901588094,0.268030405508375,
-4.42035895749369));
#364061=CARTESIAN_POINT('Ctrl Pts',(1.21410782431093,-0.0484964950687469,
-4.48098935724673));
#364062=CARTESIAN_POINT('Ctrl Pts',(1.15951315008879,-0.361626396644902,
-4.54161761073803));
#364063=CARTESIAN_POINT('Ctrl Pts',(1.02725603829703,-0.648203803698725,
-4.6015889574937));
#364064=CARTESIAN_POINT('Ctrl Pts',(0.824211675135013,-0.892796076188798,
-4.66221935724673));
#364065=CARTESIAN_POINT('Ctrl Pts',(0.564191133979094,-1.07560808862644,
-4.722847610738));
#364066=CARTESIAN_POINT('Ctrl Pts',(0.268030405508374,-1.18472901588094,
-4.7828189574937));
#364067=CARTESIAN_POINT('Ctrl Pts',(-0.04849649506876,-1.21410782431095,
-4.84344935724668));
#364068=CARTESIAN_POINT('Ctrl Pts',(-0.361626396644897,-1.15951315008877,
-4.90407761073806));
#364069=CARTESIAN_POINT('Ctrl Pts',(-0.648203803698715,-1.02725603829702,
-4.96404895749372));
#364070=CARTESIAN_POINT('Ctrl Pts',(-0.892796076188803,-0.824211675135015,
-5.02467935724671));
#364071=CARTESIAN_POINT('Ctrl Pts',(-1.07560808862644,-0.564191133979088,
-5.085307610738));
#364072=CARTESIAN_POINT('Ctrl Pts',(-1.18472901588092,-0.268030405508372,
-5.14527895749374));
#364073=CARTESIAN_POINT('Ctrl Pts',(-1.21410782431095,0.0484964950687572,
-5.20590935724669));
#364074=CARTESIAN_POINT('Ctrl Pts',(-1.1595131500888,0.361626396644921,
-5.26653761073799));
#364075=CARTESIAN_POINT('Ctrl Pts',(-1.02725603829702,0.64820380369872,
-5.32650895749373));
#364076=CARTESIAN_POINT('Ctrl Pts',(-0.824211675135014,0.892796076188816,
-5.38713935724669));
#364077=CARTESIAN_POINT('Ctrl Pts',(-0.564191133979076,1.07560808862641,
-5.44776761073806));
#364078=CARTESIAN_POINT('Ctrl Pts',(-0.268030405508379,1.18472901588095,
-5.50773895749365));
#364079=CARTESIAN_POINT('Ctrl Pts',(0.0484964950687955,1.21410782431095,
-5.56836935724668));
#364080=CARTESIAN_POINT('Ctrl Pts',(0.361626396644923,1.15951315008874,
-5.62899761073811));
#364081=CARTESIAN_POINT('Ctrl Pts',(0.648203803698529,1.02725603829711,
-5.68896895749371));
#364082=CARTESIAN_POINT('Ctrl Pts',(0.892796076189156,0.824211675134774,
-5.74959935724652));
#364083=CARTESIAN_POINT('Ctrl Pts',(1.07560808862635,0.564191133979143,
-5.81022761073827));
#364084=CARTESIAN_POINT('Ctrl Pts',(1.18472901588091,0.268030405509044,
-5.87019895749336));
#364085=CARTESIAN_POINT('Ctrl Pts',(1.2141078243105,-0.0484964950705043,
-5.93082935724695));
#364086=CARTESIAN_POINT('Ctrl Pts',(1.15951315009036,-0.361626396638523,
-5.99145761073686));
#364087=CARTESIAN_POINT('Ctrl Pts',(1.02725603828656,-0.648203803720622,
-6.05142895750248));
#364088=CARTESIAN_POINT('Ctrl Pts',(0.824211675164934,-0.892796076174764,
-6.11205935720599));
#364089=CARTESIAN_POINT('Ctrl Pts',(0.564191134059871,-1.07560808852829,
-6.17268761076101));
#364090=CARTESIAN_POINT('Ctrl Pts',(0.268030404959908,-1.18472901600022,
-6.23265895786053));
#364091=CARTESIAN_POINT('Ctrl Pts',(-0.048496494303855,-1.21410782509991,
-6.29328935527559));
#364092=CARTESIAN_POINT('Ctrl Pts',(-0.361626395111129,-1.15951314891753,
-6.35391761278417));
#364093=CARTESIAN_POINT('Ctrl Pts',(-0.648203807785757,-1.02725603400328,
-6.41388896506857));
#364094=CARTESIAN_POINT('Ctrl Pts',(-0.892796086148053,-0.82421169457497,
-6.47451931057689));
#364095=CARTESIAN_POINT('Ctrl Pts',(-1.0756080601232,-0.564191117561312,
-6.53514766561185));
#364096=CARTESIAN_POINT('Ctrl Pts',(-1.18472898053544,-0.268030410347432,
-6.59511906407632));
#364097=CARTESIAN_POINT('Ctrl Pts',(-1.21410817056974,0.0484965775982433,
-6.65574860156863));
#364098=CARTESIAN_POINT('Ctrl Pts',(-1.15951264802113,0.361626359829526,
-6.71637855817043));
#364099=CARTESIAN_POINT('Ctrl Pts',(-1.02725631549215,0.648202679709777,
-6.77634998994504));
#364100=CARTESIAN_POINT('Ctrl Pts',(-0.824212514048729,0.89279989750689,
-6.83697046026166));
#364101=CARTESIAN_POINT('Ctrl Pts',(-0.564185827571163,1.07561000588125,
-6.89761936594616));
#364102=CARTESIAN_POINT('Ctrl Pts',(-0.268055236457238,1.1847006164406,
-6.95758396792716));
#364103=CARTESIAN_POINT('Ctrl Pts',(0.0485472352404887,1.2142038916925,
-7.01813896161907));
#364104=CARTESIAN_POINT('Ctrl Pts',(0.361655804485534,1.15924149264237,
-7.07893382111904));
#364105=CARTESIAN_POINT('Ctrl Pts',(0.6478968782727,1.02825270748,-7.1387952204064));
#364106=CARTESIAN_POINT('Ctrl Pts',(0.893414088159582,0.820656810820771,
-7.19914743650299));
#364107=CARTESIAN_POINT('Ctrl Pts',(1.07501647976632,0.576321349623175,
-7.26054245691513));
#364108=CARTESIAN_POINT('Ctrl Pts',(1.18621324528802,0.224452404214759,
-7.3192609169548));
#364109=CARTESIAN_POINT('Ctrl Pts',(1.20016374408797,0.152327073866745,
-7.36128002094695));
#364110=CARTESIAN_POINT('Ctrl Pts',(1.20016374408796,-0.0349890780536599,
-7.37928962624155));
#364111=CARTESIAN_POINT('Ctrl Pts',(1.19994860179671,0.0349330361207006,
-2.22019720516939));
#364112=CARTESIAN_POINT('Ctrl Pts',(1.19994860179671,-0.126746617464705,
-2.23574197648456));
#364113=CARTESIAN_POINT('Ctrl Pts',(1.18628451104366,-0.235287042882826,
-2.2810964912132));
#364114=CARTESIAN_POINT('Ctrl Pts',(1.07477771342961,-0.573169099315595,
-2.33867755519319));
#364115=CARTESIAN_POINT('Ctrl Pts',(0.893209191596192,-0.821391071780957,
-2.40041325450729));
#364116=CARTESIAN_POINT('Ctrl Pts',(0.647719578695754,-1.02788019949386,
-2.46067439994995));
#364117=CARTESIAN_POINT('Ctrl Pts',(0.361523604188232,-1.15911171219588,
-2.52056034931245));
#364118=CARTESIAN_POINT('Ctrl Pts',(0.0484713603287608,-1.21397018964645,
-2.58134810525369));
#364119=CARTESIAN_POINT('Ctrl Pts',(-0.26807499252822,-1.18447453220047,
-2.64190541780525));
#364120=CARTESIAN_POINT('Ctrl Pts',(-0.564145022724671,-1.07538119354467,
-2.70186948165707));
#364121=CARTESIAN_POINT('Ctrl Pts',(-0.82411227040745,-0.892592747940269,
-2.76251800818134));
#364122=CARTESIAN_POINT('Ctrl Pts',(-1.02710741719481,-0.648025648702113,
-2.82313903087394));
#364123=CARTESIAN_POINT('Ctrl Pts',(-1.15932278442025,-0.361494315792975,
-2.88311038111178));
#364124=CARTESIAN_POINT('Ctrl Pts',(-1.21389060301799,-0.0484207535259056,
-2.94373983918878));
#364125=CARTESIAN_POINT('Ctrl Pts',(-1.18449856839689,0.268050248144059,
-3.00436996521972));
#364126=CARTESIAN_POINT('Ctrl Pts',(-1.0753804241319,0.564150242879215,
-3.06434127064474));
#364127=CARTESIAN_POINT('Ctrl Pts',(-0.892588631186338,0.824111463629319,
-3.12496913072614));
#364128=CARTESIAN_POINT('Ctrl Pts',(-0.648026852820059,1.02710713661446,
-3.18560006416148));
#364129=CARTESIAN_POINT('Ctrl Pts',(-0.361494335707408,1.15932328272349,
-3.24557132342766));
#364130=CARTESIAN_POINT('Ctrl Pts',(-0.0484206753242147,1.21389025844596,
-3.30619908602272));
#364131=CARTESIAN_POINT('Ctrl Pts',(0.268050244650624,1.18449860355023,
-3.36683007137514));
#364132=CARTESIAN_POINT('Ctrl Pts',(0.564150258467979,1.07538045277468,
-3.42680132544561));
#364133=CARTESIAN_POINT('Ctrl Pts',(0.824111444426381,0.892588621200653,
-3.48742908409296));
#364134=CARTESIAN_POINT('Ctrl Pts',(1.02710714086036,0.648026848734914,
-3.54806007173318));
#364135=CARTESIAN_POINT('Ctrl Pts',(1.15932328389686,0.361494337262554,
-3.60803132546964));
#364136=CARTESIAN_POINT('Ctrl Pts',(1.21389025765669,0.0484206760863054,
-3.66865908405205));
#364137=CARTESIAN_POINT('Ctrl Pts',(1.18449860343075,-0.268050245199621,
-3.72929007174227));
#364138=CARTESIAN_POINT('Ctrl Pts',(1.07538045287309,-0.564150258386447,
-3.78926132546809));
#364139=CARTESIAN_POINT('Ctrl Pts',(0.892588621215019,-0.824111444396376,
-3.84988908405249));
#364140=CARTESIAN_POINT('Ctrl Pts',(0.648026848712835,-1.02710714087089,
-3.91052007174198));
#364141=CARTESIAN_POINT('Ctrl Pts',(0.361494337268959,-1.15932328389524,
-3.97049132546837));
#364142=CARTESIAN_POINT('Ctrl Pts',(0.0484206760845926,-1.21389025765713,
-4.03111908405232));
#364143=CARTESIAN_POINT('Ctrl Pts',(-0.268050245198952,-1.18449860343081,
-4.09175007174202));
#364144=CARTESIAN_POINT('Ctrl Pts',(-0.564150258386389,-1.07538045287319,
-4.15172132546838));
#364145=CARTESIAN_POINT('Ctrl Pts',(-0.82411144439661,-0.892588621214665,
-4.2123490840523));
#364146=CARTESIAN_POINT('Ctrl Pts',(-1.0271071408708,-0.648026848713027,
-4.27298007174198));
#364147=CARTESIAN_POINT('Ctrl Pts',(-1.15932328389526,-0.361494337268938,
-4.33295132546841));
#364148=CARTESIAN_POINT('Ctrl Pts',(-1.21389025765712,-0.0484206760845532,
-4.39357908405229));
#364149=CARTESIAN_POINT('Ctrl Pts',(-1.1844986034308,0.268050245198939,
-4.45421007174199));
#364150=CARTESIAN_POINT('Ctrl Pts',(-1.07538045287319,0.564150258386394,
-4.51418132546839));
#364151=CARTESIAN_POINT('Ctrl Pts',(-0.892588621214658,0.82411144439661,
-4.5748090840523));
#364152=CARTESIAN_POINT('Ctrl Pts',(-0.648026848713022,1.0271071408708,
-4.63544007174198));
#364153=CARTESIAN_POINT('Ctrl Pts',(-0.361494337268941,1.15932328389527,
-4.69541132546844));
#364154=CARTESIAN_POINT('Ctrl Pts',(-0.0484206760845442,1.21389025765711,
-4.75603908405227));
#364155=CARTESIAN_POINT('Ctrl Pts',(0.268050245198942,1.18449860343081,
-4.81667007174201));
#364156=CARTESIAN_POINT('Ctrl Pts',(0.564150258386395,1.07538045287318,
-4.87664132546839));
#364157=CARTESIAN_POINT('Ctrl Pts',(0.824111444396615,0.892588621214655,
-4.9372690840523));
#364158=CARTESIAN_POINT('Ctrl Pts',(1.02710714087079,0.648026848713006,
-4.99790007174195));
#364159=CARTESIAN_POINT('Ctrl Pts',(1.15932328389525,0.361494337268927,
-5.0578713254684));
#364160=CARTESIAN_POINT('Ctrl Pts',(1.21389025765711,0.0484206760845428,
-5.11849908405229));
#364161=CARTESIAN_POINT('Ctrl Pts',(1.1844986034308,-0.268050245198941,
-5.179130071742));
#364162=CARTESIAN_POINT('Ctrl Pts',(1.07538045287319,-0.5641502583864,-5.2391013254684));
#364163=CARTESIAN_POINT('Ctrl Pts',(0.892588621214648,-0.824111444396615,
-5.29972908405229));
#364164=CARTESIAN_POINT('Ctrl Pts',(0.648026848713012,-1.0271071408708,
-5.36036007174197));
#364165=CARTESIAN_POINT('Ctrl Pts',(0.361494337268925,-1.15932328389526,
-5.42033132546841));
#364166=CARTESIAN_POINT('Ctrl Pts',(0.0484206760845338,-1.21389025765709,
-5.48095908405224));
#364167=CARTESIAN_POINT('Ctrl Pts',(-0.268050245198938,-1.18449860343081,
-5.54159007174203));
#364168=CARTESIAN_POINT('Ctrl Pts',(-0.564150258386406,-1.0753804528732,
-5.60156132546843));
#364169=CARTESIAN_POINT('Ctrl Pts',(-0.824111444396613,-0.89258862121464,
-5.66218908405228));
#364170=CARTESIAN_POINT('Ctrl Pts',(-1.02710714087079,-0.648026848713008,
-5.72282007174197));
#364171=CARTESIAN_POINT('Ctrl Pts',(-1.15932328389528,-0.36149433726893,
-5.78279132546845));
#364172=CARTESIAN_POINT('Ctrl Pts',(-1.2138902576571,-0.0484206760845329,
-5.84341908405225));
#364173=CARTESIAN_POINT('Ctrl Pts',(-1.18449860343078,0.268050245198954,
-5.90405007174196));
#364174=CARTESIAN_POINT('Ctrl Pts',(-1.07538045287319,0.564150258386408,
-5.96402132546844));
#364175=CARTESIAN_POINT('Ctrl Pts',(-0.892588621214629,0.824111444396606,
-6.02464908405225));
#364176=CARTESIAN_POINT('Ctrl Pts',(-0.64802684871302,1.02710714087081,
-6.08528007174203));
#364177=CARTESIAN_POINT('Ctrl Pts',(-0.361494337268917,1.15932328389523,
-6.14525132546836));
#364178=CARTESIAN_POINT('Ctrl Pts',(-0.048420676084498,1.21389025765709,
-6.20587908405224));
#364179=CARTESIAN_POINT('Ctrl Pts',(0.268050245198975,1.18449860343083,
-6.26651007174208));
#364180=CARTESIAN_POINT('Ctrl Pts',(0.564150258386226,1.07538045287327,
-6.32648132546841));
#364181=CARTESIAN_POINT('Ctrl Pts',(0.824111444396827,0.892588621214275,
-6.38710908405208));
#364182=CARTESIAN_POINT('Ctrl Pts',(1.0271071408709,0.648026848713156,-6.44774007174223));
#364183=CARTESIAN_POINT('Ctrl Pts',(1.159323283895,0.361494337269589,-6.50771132546807));
#364184=CARTESIAN_POINT('Ctrl Pts',(1.21389025765673,0.0484206760826282,
-6.56833908405251));
#364185=CARTESIAN_POINT('Ctrl Pts',(1.18449860343187,-0.268050245192022,
-6.62897007174084));
#364186=CARTESIAN_POINT('Ctrl Pts',(1.07538045286828,-0.564150258411146,
-6.68894132547714));
#364187=CARTESIAN_POINT('Ctrl Pts',(0.892588621213993,-0.824111444364615,
-6.74956908401155));
#364188=CARTESIAN_POINT('Ctrl Pts',(0.648026848838496,-1.0271071407854,
-6.81020007176602));
#364189=CARTESIAN_POINT('Ctrl Pts',(0.361494336755823,-1.1593232842844,
-6.87017132583052));
#364190=CARTESIAN_POINT('Ctrl Pts',(0.0484206766338695,-1.2138902567815,
-6.93079908208711));
#364191=CARTESIAN_POINT('Ctrl Pts',(-0.268050243328471,-1.18449860442843,
-6.99143007381518));
#364192=CARTESIAN_POINT('Ctrl Pts',(-0.564150266443273,-1.07538045302616,
-7.05140133291083));
#364193=CARTESIAN_POINT('Ctrl Pts',(-0.824111428662813,-0.892588609834598,
-7.11202903755537));
#364194=CARTESIAN_POINT('Ctrl Pts',(-1.02710714802879,-0.648026871740004,
-7.17266012714546));
#364195=CARTESIAN_POINT('Ctrl Pts',(-1.15932333812035,-0.361494339370128,
-7.23263142938285));
#364196=CARTESIAN_POINT('Ctrl Pts',(-1.21388994830272,-0.048420558641127,
-7.29325833250989));
#364197=CARTESIAN_POINT('Ctrl Pts',(-1.18449897688191,0.268050252868152,
-7.3538910230542));
#364198=CARTESIAN_POINT('Ctrl Pts',(-1.07538131032931,0.564149776786355,
-7.41386233272661));
#364199=CARTESIAN_POINT('Ctrl Pts',(-0.89258382755218,0.824110299740277,
-7.47448020435212));
#364200=CARTESIAN_POINT('Ctrl Pts',(-0.648027824318076,1.02711576339274,
-7.53513199456933));
#364201=CARTESIAN_POINT('Ctrl Pts',(-0.361519103800307,1.1593054263198,
-7.59509558925458));
#364202=CARTESIAN_POINT('Ctrl Pts',(-0.048363558710048,1.21390597518738,
-7.65565075634608));
#364203=CARTESIAN_POINT('Ctrl Pts',(0.268072537684821,1.18437146807072,
-7.71644050362745));
#364204=CARTESIAN_POINT('Ctrl Pts',(0.563930411939142,1.07613883654808,
-7.77632820376135));
#364205=CARTESIAN_POINT('Ctrl Pts',(0.82426225220675,0.889715887308659,
-7.83657609568004));
#364206=CARTESIAN_POINT('Ctrl Pts',(1.02783344969258,0.657090690457504,
-7.89836582380498));
#364207=CARTESIAN_POINT('Ctrl Pts',(1.15670010462145,0.329911052415485,
-7.95561053869555));
#364208=CARTESIAN_POINT('Ctrl Pts',(1.19983645566974,0.222219960564689,
-8.00127996772839));
#364209=CARTESIAN_POINT('Ctrl Pts',(1.19983645566973,0.0349038086442839,
-8.01928957302298));
#364210=CARTESIAN_POINT('Ctrl Pts',(1.99994859520949,0.0349419760186855,
-2.22027906663631));
#364211=CARTESIAN_POINT('Ctrl Pts',(1.99994859520949,-0.133161143166691,
-2.23644142527053));
#364212=CARTESIAN_POINT('Ctrl Pts',(1.96833139354662,-0.472425718114294,
-2.28062587414611));
#364213=CARTESIAN_POINT('Ctrl Pts',(1.77549751488388,-0.970378153502274,
-2.33932132964638));
#364214=CARTESIAN_POINT('Ctrl Pts',(1.46486827473653,-1.39599810161593,
-2.40041168228136));
#364215=CARTESIAN_POINT('Ctrl Pts',(1.0532724675317,-1.72756949816,-2.46064650153962));
#364216=CARTESIAN_POINT('Ctrl Pts',(0.570253827701872,-1.94116844962337,
-2.52097328730337));
#364217=CARTESIAN_POINT('Ctrl Pts',(0.0484505622703552,-2.02298787581022,
-2.58147196284819));
#364218=CARTESIAN_POINT('Ctrl Pts',(-0.476762817249676,-1.96636546213765,
-2.64190473727344));
#364219=CARTESIAN_POINT('Ctrl Pts',(-0.969389646094711,-1.7758542783469,
-2.70222141276452));
#364220=CARTESIAN_POINT('Ctrl Pts',(-1.39619412835269,-1.46471035101601,
-2.76268238970025));
#364221=CARTESIAN_POINT('Ctrl Pts',(-1.72755848446788,-1.05330968911041,
-2.8231370123091));
#364222=CARTESIAN_POINT('Ctrl Pts',(-1.94118200928605,-0.570259037663673,
-2.88345449584336));
#364223=CARTESIAN_POINT('Ctrl Pts',(-2.02296215046454,-0.0484473116516587,
-2.94390972032538));
#364224=CARTESIAN_POINT('Ctrl Pts',(-1.96637109382515,0.476765855935366,
-3.00436740295728));
#364225=CARTESIAN_POINT('Ctrl Pts',(-1.77585739520295,0.969389009874219,
-3.06468474103924));
#364226=CARTESIAN_POINT('Ctrl Pts',(-1.46470740175196,1.39619269138418,
-3.12513949735647));
#364227=CARTESIAN_POINT('Ctrl Pts',(-1.05331000180424,1.72755870986409,
-3.18559743702838));
#364228=CARTESIAN_POINT('Ctrl Pts',(-0.570259275444307,1.94118238224882,
-3.2459147561141));
#364229=CARTESIAN_POINT('Ctrl Pts',(-0.0484472107178668,2.02296183497224,
-3.30636948355066));
#364230=CARTESIAN_POINT('Ctrl Pts',(0.476765831354286,1.96637112545875,
-3.36682743921798));
#364231=CARTESIAN_POINT('Ctrl Pts',(0.969389026744113,1.77585742843582,
-3.42714475673536));
#364232=CARTESIAN_POINT('Ctrl Pts',(1.39619267971627,1.46470738191116,-3.48759948296635));
#364233=CARTESIAN_POINT('Ctrl Pts',(1.72755870948907,1.05331000492523,-3.54805743931225));
#364234=CARTESIAN_POINT('Ctrl Pts',(1.9411823845861,0.570259275622033,-3.60837475674778));
#364235=CARTESIAN_POINT('Ctrl Pts',(2.02296183383815,0.0484472105365179,
-3.66882948295392));
#364236=CARTESIAN_POINT('Ctrl Pts',(1.96637112555601,-0.476765831198158,
-3.72928743931407));
#364237=CARTESIAN_POINT('Ctrl Pts',(1.77585742848668,-0.969389026837108,
-3.78960475674772));
#364238=CARTESIAN_POINT('Ctrl Pts',(1.46470738188885,-1.39619267968778,
-3.85005948295395));
#364239=CARTESIAN_POINT('Ctrl Pts',(1.05331000493188,-1.72755870948857,
-3.910517439314));
#364240=CARTESIAN_POINT('Ctrl Pts',(0.570259275619007,-1.9411823845877,
-3.97083475674782));
#364241=CARTESIAN_POINT('Ctrl Pts',(0.0484472105373659,-2.02296183383781,
-4.03128948295388));
#364242=CARTESIAN_POINT('Ctrl Pts',(-0.476765831198311,-1.96637112555626,
-4.09174743931402));
#364243=CARTESIAN_POINT('Ctrl Pts',(-0.969389026837092,-1.77585742848654,
-4.15206475674782));
#364244=CARTESIAN_POINT('Ctrl Pts',(-1.39619267968775,-1.46470738188883,
-4.21251948295388));
#364245=CARTESIAN_POINT('Ctrl Pts',(-1.72755870948862,-1.05331000493188,
-4.27297743931401));
#364246=CARTESIAN_POINT('Ctrl Pts',(-1.94118238458768,-0.570259275619005,
-4.33329475674783));
#364247=CARTESIAN_POINT('Ctrl Pts',(-2.0229618338378,-0.0484472105373586,
-4.39374948295387));
#364248=CARTESIAN_POINT('Ctrl Pts',(-1.96637112555625,0.476765831198322,
-4.45420743931402));
#364249=CARTESIAN_POINT('Ctrl Pts',(-1.77585742848654,0.969389026837096,
-4.51452475674782));
#364250=CARTESIAN_POINT('Ctrl Pts',(-1.46470738188882,1.39619267968775,
-4.57497948295388));
#364251=CARTESIAN_POINT('Ctrl Pts',(-1.05331000493187,1.72755870948862,
-4.63543743931401));
#364252=CARTESIAN_POINT('Ctrl Pts',(-0.570259275619004,1.9411823845877,
-4.69575475674784));
#364253=CARTESIAN_POINT('Ctrl Pts',(-0.0484472105373471,2.0229618338378,
-4.75620948295387));
#364254=CARTESIAN_POINT('Ctrl Pts',(0.476765831198326,1.96637112555626,
-4.81666743931402));
#364255=CARTESIAN_POINT('Ctrl Pts',(0.969389026837101,1.77585742848653,
-4.87698475674782));
#364256=CARTESIAN_POINT('Ctrl Pts',(1.39619267968776,1.46470738188882,-4.93743948295388));
#364257=CARTESIAN_POINT('Ctrl Pts',(1.72755870948861,1.05331000493185,-4.997897439314));
#364258=CARTESIAN_POINT('Ctrl Pts',(1.94118238458768,0.570259275618993,
-5.05821475674782));
#364259=CARTESIAN_POINT('Ctrl Pts',(2.0229618338378,0.0484472105373451,
-5.11866948295387));
#364260=CARTESIAN_POINT('Ctrl Pts',(1.96637112555625,-0.476765831198331,
-5.17912743931402));
#364261=CARTESIAN_POINT('Ctrl Pts',(1.77585742848654,-0.969389026837107,
-5.23944475674783));
#364262=CARTESIAN_POINT('Ctrl Pts',(1.46470738188881,-1.39619267968776,
-5.29989948295387));
#364263=CARTESIAN_POINT('Ctrl Pts',(1.05331000493185,-1.72755870948862,
-5.36035743931401));
#364264=CARTESIAN_POINT('Ctrl Pts',(0.57025927561899,-1.94118238458768,
-5.42067475674783));
#364265=CARTESIAN_POINT('Ctrl Pts',(0.0484472105373359,-2.02296183383778,
-5.48112948295386));
#364266=CARTESIAN_POINT('Ctrl Pts',(-0.476765831198329,-1.96637112555626,
-5.54158743931402));
#364267=CARTESIAN_POINT('Ctrl Pts',(-0.96938902683712,-1.77585742848655,
-5.60190475674783));
#364268=CARTESIAN_POINT('Ctrl Pts',(-1.39619267968776,-1.4647073818888,
-5.66235948295387));
#364269=CARTESIAN_POINT('Ctrl Pts',(-1.72755870948862,-1.05331000493185,
-5.722817439314));
#364270=CARTESIAN_POINT('Ctrl Pts',(-1.9411823845877,-0.570259275618991,
-5.78313475674784));
#364271=CARTESIAN_POINT('Ctrl Pts',(-2.02296183383779,-0.0484472105373294,
-5.84358948295386));
#364272=CARTESIAN_POINT('Ctrl Pts',(-1.96637112555623,0.476765831198343,
-5.904047439314));
#364273=CARTESIAN_POINT('Ctrl Pts',(-1.77585742848654,0.969389026837124,
-5.96436475674784));
#364274=CARTESIAN_POINT('Ctrl Pts',(-1.46470738188879,1.39619267968775,
-6.02481948295386));
#364275=CARTESIAN_POINT('Ctrl Pts',(-1.05331000493186,1.72755870948864,
-6.08527743931403));
#364276=CARTESIAN_POINT('Ctrl Pts',(-0.57025927561896,1.94118238458767,
-6.14559475674781));
#364277=CARTESIAN_POINT('Ctrl Pts',(-0.0484472105373227,2.02296183383776,
-6.20604948295386));
#364278=CARTESIAN_POINT('Ctrl Pts',(0.476765831198343,1.96637112555631,
-6.26650743931404));
#364279=CARTESIAN_POINT('Ctrl Pts',(0.969389026837138,1.77585742848649,
-6.32682475674784));
#364280=CARTESIAN_POINT('Ctrl Pts',(1.39619267968763,1.4647073818887,-6.3872794829538));
#364281=CARTESIAN_POINT('Ctrl Pts',(1.72755870948896,1.05331000493196,-6.4477374393141));
#364282=CARTESIAN_POINT('Ctrl Pts',(1.94118238458724,0.570259275618813,
-6.50805475674775));
#364283=CARTESIAN_POINT('Ctrl Pts',(2.0229618338382,0.0484472105380158,
-6.56850948295382));
#364284=CARTESIAN_POINT('Ctrl Pts',(1.96637112555413,-0.47676583120083,
-6.62896743931409));
#364285=CARTESIAN_POINT('Ctrl Pts',(1.77585742849251,-0.969389026833344,
-6.68928475674954));
#364286=CARTESIAN_POINT('Ctrl Pts',(1.46470738188697,-1.39619267969199,
-6.74973948294137));
#364287=CARTESIAN_POINT('Ctrl Pts',(1.05331000488233,-1.72755870945149,
-6.81019743932769));
#364288=CARTESIAN_POINT('Ctrl Pts',(0.570259275809968,-1.94118238475938,
-6.87051475683913));
#364289=CARTESIAN_POINT('Ctrl Pts',(0.0484472101488399,-2.02296183330866,
-6.93096948236246));
#364290=CARTESIAN_POINT('Ctrl Pts',(-0.476765830732716,-1.96637112538019,
-6.99142743997978));
#364291=CARTESIAN_POINT('Ctrl Pts',(-0.969389027651612,-1.775857433288,
-7.05174475889683));
#364292=CARTESIAN_POINT('Ctrl Pts',(-1.39619267380615,-1.46470736293583,
-7.11219946872276));
#364293=CARTESIAN_POINT('Ctrl Pts',(-1.72755871231312,-1.05331002647757,
-7.1726574556236));
#364294=CARTESIAN_POINT('Ctrl Pts',(-1.94118244199894,-0.570259298778077,
-7.23297479041701));
#364295=CARTESIAN_POINT('Ctrl Pts',(-2.02296149561613,-0.0484470734163606,
-7.29342924947211));
#364296=CARTESIAN_POINT('Ctrl Pts',(-1.96637162260829,0.47676563992917,
-7.35388770608518));
#364297=CARTESIAN_POINT('Ctrl Pts',(-1.77585778550465,0.969389377563547,
-7.41420515419699));
#364298=CARTESIAN_POINT('Ctrl Pts',(-1.46470321414872,1.39619055347437,
-7.4746566054593));
#364299=CARTESIAN_POINT('Ctrl Pts',(-1.05331679189158,1.72756279918536,
-7.53512091909894));
#364300=CARTESIAN_POINT('Ctrl Pts',(-0.570256351317271,1.94118541096824,
-7.5954368568002));
#364301=CARTESIAN_POINT('Ctrl Pts',(-0.0484373346474795,2.02291433148142,
-7.65586848775589));
#364302=CARTESIAN_POINT('Ctrl Pts',(0.476753357889169,1.96647633924905,
-7.7163654145941));
#364303=CARTESIAN_POINT('Ctrl Pts',(0.969439733353148,1.77572407380791,
-7.7767079034587));
#364304=CARTESIAN_POINT('Ctrl Pts',(1.39587962475789,1.46484458461224,-7.83687735653918));
#364305=CARTESIAN_POINT('Ctrl Pts',(1.72854436163452,1.05253719801599,-7.89821617217114));
#364306=CARTESIAN_POINT('Ctrl Pts',(1.93848294702123,0.574209674581668,
-7.95584767975511));
#364307=CARTESIAN_POINT('Ctrl Pts',(1.99983638908382,0.21585245779268,-8.0021551741418));
#364308=CARTESIAN_POINT('Ctrl Pts',(1.99983638908381,0.0349322317806574,
-8.0195498399348));
#364309=CARTESIAN_POINT('Ctrl Pts',(2.79994858862227,0.0349509159166703,
-2.22036092810323));
#364310=CARTESIAN_POINT('Ctrl Pts',(2.79994858862227,-0.139575668868676,
-2.2371408740565));
#364311=CARTESIAN_POINT('Ctrl Pts',(2.75037827604958,-0.709564393345761,
-2.28015525707901));
#364312=CARTESIAN_POINT('Ctrl Pts',(2.47621731633814,-1.36758720768895,
-2.33996510409957));
#364313=CARTESIAN_POINT('Ctrl Pts',(2.03652735787686,-1.97060513145091,
-2.40041011005543));
#364314=CARTESIAN_POINT('Ctrl Pts',(1.45882535636765,-2.42725879682614,
-2.46061860312929));
#364315=CARTESIAN_POINT('Ctrl Pts',(0.778984051215511,-2.72322518705085,
-2.52138622529428));
#364316=CARTESIAN_POINT('Ctrl Pts',(0.0484297642119496,-2.83200556197398,
-2.58159582044269));
#364317=CARTESIAN_POINT('Ctrl Pts',(-0.685450641971131,-2.74825639207482,
-2.64190405674164));
#364318=CARTESIAN_POINT('Ctrl Pts',(-1.37463426946475,-2.47632736314912,
-2.70257334387197));
#364319=CARTESIAN_POINT('Ctrl Pts',(-1.96827598629794,-2.03682795409175,
-2.76284677121916));
#364320=CARTESIAN_POINT('Ctrl Pts',(-2.42800955174095,-1.45859372951871,
-2.82313499374427));
#364321=CARTESIAN_POINT('Ctrl Pts',(-2.72304123415184,-0.779023759534372,
-2.88379861057494));
#364322=CARTESIAN_POINT('Ctrl Pts',(-2.8320336979111,-0.048473869777412,
-2.94407960146198));
#364323=CARTESIAN_POINT('Ctrl Pts',(-2.74824361925341,0.685481463726674,
-3.00436484069483));
#364324=CARTESIAN_POINT('Ctrl Pts',(-2.47633436627399,1.37462777686922,
-3.06502821143375));
#364325=CARTESIAN_POINT('Ctrl Pts',(-2.03682617231757,1.96827391913905,
-3.1253098639868));
#364326=CARTESIAN_POINT('Ctrl Pts',(-1.45859315078841,2.42801028311372,
-3.18559480989526));
#364327=CARTESIAN_POINT('Ctrl Pts',(-0.779024215181206,2.72304148177415,
-3.24625818880055));
#364328=CARTESIAN_POINT('Ctrl Pts',(-0.048473746111519,2.83203341149851,
-3.30653988107861));
#364329=CARTESIAN_POINT('Ctrl Pts',(0.685481418057947,2.74824364736727,
-3.36682480706082));
#364330=CARTESIAN_POINT('Ctrl Pts',(1.37462779502025,2.47633440409695,-3.42748818802511));
#364331=CARTESIAN_POINT('Ctrl Pts',(1.96827391500616,2.03682614262167,-3.48776988183974));
#364332=CARTESIAN_POINT('Ctrl Pts',(2.42801027811778,1.45859316111554,-3.54805480689131));
#364333=CARTESIAN_POINT('Ctrl Pts',(2.72304148527533,0.779024213981512,
-3.60871818802593));
#364334=CARTESIAN_POINT('Ctrl Pts',(2.83203341001962,0.0484737449867304,
-3.66899988185579));
#364335=CARTESIAN_POINT('Ctrl Pts',(2.74824364768127,-0.685481417196696,
-3.72928480688587));
#364336=CARTESIAN_POINT('Ctrl Pts',(2.47633440410028,-1.37462779528777,
-3.78994818802735));
#364337=CARTESIAN_POINT('Ctrl Pts',(2.03682614256268,-1.96827391497919,
-3.85022988185542));
#364338=CARTESIAN_POINT('Ctrl Pts',(1.45859316115093,-2.42801027810626,
-3.91051480688602));
#364339=CARTESIAN_POINT('Ctrl Pts',(0.779024213969054,-2.72304148528015,
-3.97117818802726));
#364340=CARTESIAN_POINT('Ctrl Pts',(0.0484737449901392,-2.83203341001849,
-4.03145988185545));
#364341=CARTESIAN_POINT('Ctrl Pts',(-0.685481417197671,-2.74824364768172,
-4.09174480688602));
#364342=CARTESIAN_POINT('Ctrl Pts',(-1.3746277952878,-2.4763344040999,-4.15240818802725));
#364343=CARTESIAN_POINT('Ctrl Pts',(-1.96827391497889,-2.03682614256299,
-4.21268988185546));
#364344=CARTESIAN_POINT('Ctrl Pts',(-2.42801027810644,-1.45859316115073,
-4.27297480688604));
#364345=CARTESIAN_POINT('Ctrl Pts',(-2.72304148528011,-0.779024213969072,
-4.33363818802725));
#364346=CARTESIAN_POINT('Ctrl Pts',(-2.83203341001849,-0.0484737449901639,
-4.39391988185546));
#364347=CARTESIAN_POINT('Ctrl Pts',(-2.7482436476817,0.685481417197704,
-4.45420480688603));
#364348=CARTESIAN_POINT('Ctrl Pts',(-2.4763344040999,1.3746277952878,-4.51486818802725));
#364349=CARTESIAN_POINT('Ctrl Pts',(-2.03682614256298,1.96827391497889,
-4.57514988185546));
#364350=CARTESIAN_POINT('Ctrl Pts',(-1.45859316115072,2.42801027810644,
-4.63543480688604));
#364351=CARTESIAN_POINT('Ctrl Pts',(-0.779024213969067,2.72304148528013,
-4.69609818802723));
#364352=CARTESIAN_POINT('Ctrl Pts',(-0.04847374499015,2.83203341001848,
-4.75637988185547));
#364353=CARTESIAN_POINT('Ctrl Pts',(0.685481417197709,2.7482436476817,-4.81666480688603));
#364354=CARTESIAN_POINT('Ctrl Pts',(1.37462779528781,2.47633440409989,-4.87732818802725));
#364355=CARTESIAN_POINT('Ctrl Pts',(1.9682739149789,2.03682614256298,-4.93760988185546));
#364356=CARTESIAN_POINT('Ctrl Pts',(2.42801027810644,1.4585931611507,-4.99789480688605));
#364357=CARTESIAN_POINT('Ctrl Pts',(2.7230414852801,0.779024213969058,-5.05855818802725));
#364358=CARTESIAN_POINT('Ctrl Pts',(2.83203341001848,0.0484737449901475,
-5.11883988185546));
#364359=CARTESIAN_POINT('Ctrl Pts',(2.74824364768169,-0.685481417197721,
-5.17912480688604));
#364360=CARTESIAN_POINT('Ctrl Pts',(2.47633440409989,-1.37462779528781,
-5.23978818802725));
#364361=CARTESIAN_POINT('Ctrl Pts',(2.03682614256297,-1.9682739149789,-5.30006988185546));
#364362=CARTESIAN_POINT('Ctrl Pts',(1.45859316115069,-2.42801027810645,
-5.36035480688604));
#364363=CARTESIAN_POINT('Ctrl Pts',(0.779024213969056,-2.72304148528011,
-5.42101818802724));
#364364=CARTESIAN_POINT('Ctrl Pts',(0.0484737449901378,-2.83203341001847,
-5.48129988185548));
#364365=CARTESIAN_POINT('Ctrl Pts',(-0.685481417197721,-2.7482436476817,
-5.54158480688602));
#364366=CARTESIAN_POINT('Ctrl Pts',(-1.37462779528784,-2.4763344040999,
-5.60224818802724));
#364367=CARTESIAN_POINT('Ctrl Pts',(-1.9682739149789,-2.03682614256296,
-5.66252988185546));
#364368=CARTESIAN_POINT('Ctrl Pts',(-2.42801027810645,-1.45859316115069,
-5.72281480688604));
#364369=CARTESIAN_POINT('Ctrl Pts',(-2.72304148528013,-0.779024213969052,
-5.78347818802723));
#364370=CARTESIAN_POINT('Ctrl Pts',(-2.83203341001847,-0.0484737449901258,
-5.84375988185547));
#364371=CARTESIAN_POINT('Ctrl Pts',(-2.74824364768167,0.685481417197731,
-5.90404480688604));
#364372=CARTESIAN_POINT('Ctrl Pts',(-2.47633440409989,1.37462779528784,
-5.96470818802724));
#364373=CARTESIAN_POINT('Ctrl Pts',(-2.03682614256295,1.96827391497889,
-6.02498988185547));
#364374=CARTESIAN_POINT('Ctrl Pts',(-1.4585931611507,2.42801027810647,-6.08527480688602));
#364375=CARTESIAN_POINT('Ctrl Pts',(-0.779024213969003,2.7230414852801,
-6.14593818802726));
#364376=CARTESIAN_POINT('Ctrl Pts',(-0.0484737449901475,2.83203341001844,
-6.20621988185547));
#364377=CARTESIAN_POINT('Ctrl Pts',(0.685481417197711,2.74824364768178,
-6.266504806886));
#364378=CARTESIAN_POINT('Ctrl Pts',(1.37462779528805,2.4763344040997,-6.32716818802727));
#364379=CARTESIAN_POINT('Ctrl Pts',(1.96827391497844,2.03682614256313,-6.3874498818555));
#364380=CARTESIAN_POINT('Ctrl Pts',(2.42801027810703,1.45859316115076,-6.44773480688596));
#364381=CARTESIAN_POINT('Ctrl Pts',(2.72304148527948,0.779024213968036,
-6.50839818802743));
#364382=CARTESIAN_POINT('Ctrl Pts',(2.83203341001966,0.0484737449934034,
-6.56867988185514));
#364383=CARTESIAN_POINT('Ctrl Pts',(2.74824364767639,-0.685481417209638,
-6.62896480688735));
#364384=CARTESIAN_POINT('Ctrl Pts',(2.47633440411674,-1.37462779525554,
-6.68962818802195));
#364385=CARTESIAN_POINT('Ctrl Pts',(2.03682614255995,-1.96827391501936,
-6.74990988187118));
#364386=CARTESIAN_POINT('Ctrl Pts',(1.45859316092616,-2.42801027811759,
-6.81019480688936));
#364387=CARTESIAN_POINT('Ctrl Pts',(0.779024214864112,-2.72304148523437,
-6.87085818784773));
#364388=CARTESIAN_POINT('Ctrl Pts',(0.0484737436638102,-2.83203340983582,
-6.93113988263782));
#364389=CARTESIAN_POINT('Ctrl Pts',(-0.685481418136962,-2.74824364633194,
-6.99142480614438));
#364390=CARTESIAN_POINT('Ctrl Pts',(-1.37462778885995,-2.47633441354984,
-7.05208818488281));
#364391=CARTESIAN_POINT('Ctrl Pts',(-1.96827391894949,-2.03682611603706,
-7.11236989989014));
#364392=CARTESIAN_POINT('Ctrl Pts',(-2.42801027659746,-1.45859318121514,
-7.17265478410175));
#364393=CARTESIAN_POINT('Ctrl Pts',(-2.72304154587753,-0.779024258186026,
-7.23331815145116));
#364394=CARTESIAN_POINT('Ctrl Pts',(-2.83203304292954,-0.0484735881915938,
-7.29360016643431));
#364395=CARTESIAN_POINT('Ctrl Pts',(-2.74824426833468,0.685481026990187,
-7.35388438911616));
#364396=CARTESIAN_POINT('Ctrl Pts',(-2.47633426068,1.37462897834074,-7.41454797566736));
#364397=CARTESIAN_POINT('Ctrl Pts',(-2.03682260074525,1.96827080720847,
-7.47483300656648));
#364398=CARTESIAN_POINT('Ctrl Pts',(-1.45860575946508,2.42800983497797,
-7.53510984362855));
#364399=CARTESIAN_POINT('Ctrl Pts',(-0.778993598834234,2.72306539561668,
-7.59577812434582));
#364400=CARTESIAN_POINT('Ctrl Pts',(-0.0485111105849109,2.83192268777547,
-7.65608621916571));
#364401=CARTESIAN_POINT('Ctrl Pts',(0.685434178093518,2.74858121042738,
-7.71629032556075));
#364402=CARTESIAN_POINT('Ctrl Pts',(1.37494905476715,2.47530931106774,-7.77708760315606));
#364403=CARTESIAN_POINT('Ctrl Pts',(1.96749699730902,2.03997328191583,-7.83717861739831));
#364404=CARTESIAN_POINT('Ctrl Pts',(2.42925527357646,1.44798370557448,-7.89806652053729));
#364405=CARTESIAN_POINT('Ctrl Pts',(2.72026578942101,0.81850829674785,-7.95608482081467));
#364406=CARTESIAN_POINT('Ctrl Pts',(2.7998363224979,0.209484955020671,-8.00303038055522));
#364407=CARTESIAN_POINT('Ctrl Pts',(2.7998363224979,0.0349606549170308,
-8.01981010684662));
#364408=CARTESIAN_POINT('Ctrl Pts',(2.80005140479051,-0.0349419760186688,
-1.58036093336367));
#364409=CARTESIAN_POINT('Ctrl Pts',(2.80005140479051,-0.222315492003956,
-1.59837605395503));
#364410=CARTESIAN_POINT('Ctrl Pts',(2.7214217418683,-0.809145725726729,
-1.6432251028271));
#364411=CARTESIAN_POINT('Ctrl Pts',(2.4293855576505,-1.45019120570836,-1.70229805797781));
#364412=CARTESIAN_POINT('Ctrl Pts',(1.96768973634555,-2.03953853811049,
-1.7629395123984));
#364413=CARTESIAN_POINT('Ctrl Pts',(1.37507506915162,-2.47563743577604,
-1.8230967134397));
#364414=CARTESIAN_POINT('Ctrl Pts',(0.685513462117749,-2.74874432479135,
-1.88387667036327));
#364415=CARTESIAN_POINT('Ctrl Pts',(-0.0484811831405424,-2.83215111147164,
-1.94408480572724));
#364416=CARTESIAN_POINT('Ctrl Pts',(-0.779026681647449,-2.72327925825339,
-2.00439212797816));
#364417=CARTESIAN_POINT('Ctrl Pts',(-1.45869410662288,-2.42821024693195,
-2.0650608706179));
#364418=CARTESIAN_POINT('Ctrl Pts',(-2.03695498339253,-1.96844588111817,
-2.12533700840671));
#364419=CARTESIAN_POINT('Ctrl Pts',(-2.4765110806735,-1.3747587008243,-2.18562256240842));
#364420=CARTESIAN_POINT('Ctrl Pts',(-2.7484478409841,-0.685559860459645,
-2.24628623797644));
#364421=CARTESIAN_POINT('Ctrl Pts',(-2.83225060905395,0.048443263325025,
-2.30656987054029));
#364422=CARTESIAN_POINT('Ctrl Pts',(-2.72325825549342,0.779057613295582,
-2.36685238231703));
#364423=CARTESIAN_POINT('Ctrl Pts',(-2.42820998732486,1.45868136138043,
-2.4275158429718));
#364424=CARTESIAN_POINT('Ctrl Pts',(-1.96844920055485,2.03695852016992,
-2.48780013698524));
#364425=CARTESIAN_POINT('Ctrl Pts',(-1.37475744002027,2.4765112353038,-2.54808234902813));
#364426=CARTESIAN_POINT('Ctrl Pts',(-0.685560283084277,2.74844721593019,
-2.60874582079915));
#364427=CARTESIAN_POINT('Ctrl Pts',(0.0484434248256224,2.83225097648717,
-2.66903015426646));
#364428=CARTESIAN_POINT('Ctrl Pts',(0.7790575695397,2.72325819429533,-2.72931234606168));
#364429=CARTESIAN_POINT('Ctrl Pts',(1.45868134037711,2.42820998953338,-2.78997582004938));
#364430=CARTESIAN_POINT('Ctrl Pts',(2.0369585467678,1.96844919652417,-2.85026015503416));
#364431=CARTESIAN_POINT('Ctrl Pts',(2.47651122587901,1.37475744638445,-2.91054234588739));
#364432=CARTESIAN_POINT('Ctrl Pts',(2.74844721726047,0.68556028222042,-2.97120582005121));
#364433=CARTESIAN_POINT('Ctrl Pts',(2.8322509766735,-0.0484434261664062,
-3.03149015505023));
#364434=CARTESIAN_POINT('Ctrl Pts',(2.7232581943391,-0.779057568642653,
-3.09177234588191));
#364435=CARTESIAN_POINT('Ctrl Pts',(2.42820998952435,-1.45868134060022,
-3.15243582005264));
#364436=CARTESIAN_POINT('Ctrl Pts',(1.9684491964829,-2.03695854677124,-3.21272015504985));
#364437=CARTESIAN_POINT('Ctrl Pts',(1.37475744641701,-2.4765112258619,-3.27300234588205));
#364438=CARTESIAN_POINT('Ctrl Pts',(0.685560282208511,-2.74844721726587,
-3.33366582005255));
#364439=CARTESIAN_POINT('Ctrl Pts',(-0.0484434261631521,-2.83225097667228,
-3.39395015504989));
#364440=CARTESIAN_POINT('Ctrl Pts',(-0.779057568643627,-2.7232581943397,
-3.45423234588206));
#364441=CARTESIAN_POINT('Ctrl Pts',(-1.45868134060013,-2.42820998952376,
-3.51489582005254));
#364442=CARTESIAN_POINT('Ctrl Pts',(-2.03695854677107,-1.96844919648335,
-3.57518015504989));
#364443=CARTESIAN_POINT('Ctrl Pts',(-2.47651122586207,-1.3747574464168,
-3.63546234588207));
#364444=CARTESIAN_POINT('Ctrl Pts',(-2.74844721726579,-0.685560282208525,
-3.69612582005254));
#364445=CARTESIAN_POINT('Ctrl Pts',(-2.83225097667231,0.0484434261631291,
-3.7564101550499));
#364446=CARTESIAN_POINT('Ctrl Pts',(-2.7232581943397,0.779057568643663,
-3.81669234588207));
#364447=CARTESIAN_POINT('Ctrl Pts',(-2.42820998952376,1.45868134060013,
-3.87735582005254));
#364448=CARTESIAN_POINT('Ctrl Pts',(-1.96844919648335,2.03695854677107,
-3.9376401550499));
#364449=CARTESIAN_POINT('Ctrl Pts',(-1.37475744641679,2.47651122586208,
-3.99792234588207));
#364450=CARTESIAN_POINT('Ctrl Pts',(-0.685560282208515,2.74844721726578,
-4.05858582005252));
#364451=CARTESIAN_POINT('Ctrl Pts',(0.0484434261631405,2.83225097667232,
-4.1188701550499));
#364452=CARTESIAN_POINT('Ctrl Pts',(0.779057568643667,2.72325819433969,
-4.17915234588206));
#364453=CARTESIAN_POINT('Ctrl Pts',(1.45868134060014,2.42820998952375,-4.23981582005254));
#364454=CARTESIAN_POINT('Ctrl Pts',(2.03695854677108,1.96844919648334,-4.30010015504989));
#364455=CARTESIAN_POINT('Ctrl Pts',(2.47651122586209,1.37475744641679,-4.36038234588208));
#364456=CARTESIAN_POINT('Ctrl Pts',(2.74844721726579,0.685560282208506,
-4.42104582005254));
#364457=CARTESIAN_POINT('Ctrl Pts',(2.8322509766723,-0.0484434261631421,
-4.4813301550499));
#364458=CARTESIAN_POINT('Ctrl Pts',(2.72325819433969,-0.779057568643682,
-4.54161234588207));
#364459=CARTESIAN_POINT('Ctrl Pts',(2.42820998952373,-1.45868134060014,
-4.60227582005254));
#364460=CARTESIAN_POINT('Ctrl Pts',(1.96844919648334,-2.03695854677108,
-4.6625601550499));
#364461=CARTESIAN_POINT('Ctrl Pts',(1.37475744641678,-2.47651122586209,
-4.72284234588207));
#364462=CARTESIAN_POINT('Ctrl Pts',(0.685560282208503,-2.74844721726579,
-4.78350582005254));
#364463=CARTESIAN_POINT('Ctrl Pts',(-0.0484434261631558,-2.83225097667233,
-4.84379015504992));
#364464=CARTESIAN_POINT('Ctrl Pts',(-0.77905756864368,-2.72325819433967,
-4.90407234588205));
#364465=CARTESIAN_POINT('Ctrl Pts',(-1.45868134060014,-2.42820998952372,
-4.96473582005253));
#364466=CARTESIAN_POINT('Ctrl Pts',(-2.03695854677109,-1.96844919648334,
-5.0250201550499));
#364467=CARTESIAN_POINT('Ctrl Pts',(-2.47651122586209,-1.37475744641677,
-5.08530234588207));
#364468=CARTESIAN_POINT('Ctrl Pts',(-2.74844721726577,-0.685560282208494,
-5.14596582005252));
#364469=CARTESIAN_POINT('Ctrl Pts',(-2.83225097667232,0.0484434261631642,
-5.20625015504991));
#364470=CARTESIAN_POINT('Ctrl Pts',(-2.72325819433969,0.779057568643699,
-5.26653234588207));
#364471=CARTESIAN_POINT('Ctrl Pts',(-2.42820998952371,1.45868134060015,
-5.32719582005253));
#364472=CARTESIAN_POINT('Ctrl Pts',(-1.96844919648334,2.0369585467711,-5.38748015504991));
#364473=CARTESIAN_POINT('Ctrl Pts',(-1.37475744641676,2.47651122586207,
-5.44776234588206));
#364474=CARTESIAN_POINT('Ctrl Pts',(-0.685560282208465,2.74844721726582,
-5.50842582005256));
#364475=CARTESIAN_POINT('Ctrl Pts',(0.0484434261631459,2.8322509766723,
-5.56871015504991));
#364476=CARTESIAN_POINT('Ctrl Pts',(0.77905756864366,2.7232581943397,-5.62899234588203));
#364477=CARTESIAN_POINT('Ctrl Pts',(1.45868134060035,2.42820998952354,-5.68965582005256));
#364478=CARTESIAN_POINT('Ctrl Pts',(2.03695854677077,1.96844919648363,-5.74994015504994));
#364479=CARTESIAN_POINT('Ctrl Pts',(2.47651122586247,1.37475744641675,-5.81022234588199));
#364480=CARTESIAN_POINT('Ctrl Pts',(2.74844721726539,0.68556028220749,-5.87088582005272));
#364481=CARTESIAN_POINT('Ctrl Pts',(2.83225097667343,-0.0484434261597295,
-5.93117015504957));
#364482=CARTESIAN_POINT('Ctrl Pts',(2.72325819433488,-0.779057568656138,
-5.99145234588337));
#364483=CARTESIAN_POINT('Ctrl Pts',(2.42820998953502,-1.45868134056502,
-6.05211582004729));
#364484=CARTESIAN_POINT('Ctrl Pts',(1.96844919651089,-2.03695854682948,
-6.11240015506561));
#364485=CARTESIAN_POINT('Ctrl Pts',(1.37475744614754,-2.47651122586056,
-6.17268234588436));
#364486=CARTESIAN_POINT('Ctrl Pts',(0.685560283068197,-2.7484472169499,
-6.2333458198777));
#364487=CARTESIAN_POINT('Ctrl Pts',(-0.0484434272739145,-2.83225097815536,
-6.29363015582641));
#364488=CARTESIAN_POINT('Ctrl Pts',(-0.779057569919619,-2.72325819081683,
-6.35391234511296));
#364489=CARTESIAN_POINT('Ctrl Pts',(-1.45868133020244,-2.42820999454269,
-6.41457581704206));
#364490=CARTESIAN_POINT('Ctrl Pts',(-2.03695857643473,-1.96844920071866,
-6.47486017290601));
#364491=CARTESIAN_POINT('Ctrl Pts',(-2.47651118869187,-1.37475742725566,
-6.53514232258922));
#364492=CARTESIAN_POINT('Ctrl Pts',(-2.74844718829262,-0.685560328345768,
-6.59580578606602));
#364493=CARTESIAN_POINT('Ctrl Pts',(-2.83225126519656,0.0484435449931018,
-6.65609043578674));
#364494=CARTESIAN_POINT('Ctrl Pts',(-2.72325793947389,0.779057145346554,
-6.71637192313681));
#364495=CARTESIAN_POINT('Ctrl Pts',(-2.42820926584284,1.45868183876673,
-6.77703563697173));
#364496=CARTESIAN_POINT('Ctrl Pts',(-1.9684512872418,2.03696056375976,-6.83732324720959));
#364497=CARTESIAN_POINT('Ctrl Pts',(-1.37476376271817,2.47650348514813,
-6.89759727195412));
#364498=CARTESIAN_POINT('Ctrl Pts',(-0.685529731491166,2.74846279478609,
-6.95826629062831));
#364499=CARTESIAN_POINT('Ctrl Pts',(0.0483996833656258,2.8322123503721,
-7.01857521801487));
#364500=CARTESIAN_POINT('Ctrl Pts',(0.779017444894231,2.72348202273134,
-7.07878068295039));
#364501=CARTESIAN_POINT('Ctrl Pts',(1.45891552110071,2.42730834706515,-7.13956566066343));
#364502=CARTESIAN_POINT('Ctrl Pts',(2.03664883326185,1.97134324740292,-7.19970870776557));
#364503=CARTESIAN_POINT('Ctrl Pts',(2.47643830365019,1.36561422989075,-7.2603969994144));
#364504=CARTESIAN_POINT('Ctrl Pts',(2.74977893008757,0.719015851050413,
-7.31916157554443));
#364505=CARTESIAN_POINT('Ctrl Pts',(2.80016361091614,0.126800216505963,
-7.36426031277698));
#364506=CARTESIAN_POINT('Ctrl Pts',(2.80016361091613,-0.0349322317809129,
-7.37981016006518));
#364507=CARTESIAN_POINT('Ctrl Pts',(2.00005141137773,-0.0349509159166537,
-1.58027907189674));
#364508=CARTESIAN_POINT('Ctrl Pts',(2.00005141137773,-0.209477500702,-1.59705901785001));
#364509=CARTESIAN_POINT('Ctrl Pts',(1.93937485936534,-0.574981221086946,
-1.64398167301615));
#364510=CARTESIAN_POINT('Ctrl Pts',(1.72866575619624,-1.05218683017129,
-1.70157781695483));
#364511=CARTESIAN_POINT('Ctrl Pts',(1.39603065320521,-1.46514475575449,
-1.76296158741006));
#364512=CARTESIAN_POINT('Ctrl Pts',(0.969522180315677,-1.77589106055163,
-1.82311912419573));
#364513=CARTESIAN_POINT('Ctrl Pts',(0.476783238604109,-1.96670288995313,
-1.88346520364747));
#364514=CARTESIAN_POINT('Ctrl Pts',(-0.0484603850821368,-2.02312932285366,
-1.94396055370022));
#364515=CARTESIAN_POINT('Ctrl Pts',(-0.570338856925993,-1.94138942628423,
-2.00439291407465));
#364516=CARTESIAN_POINT('Ctrl Pts',(-1.05344948325284,-1.72773686772633,
-2.06470891120488));
#364517=CARTESIAN_POINT('Ctrl Pts',(-1.46487312544728,-1.39632835696345,
-2.1251726344757));
#364518=CARTESIAN_POINT('Ctrl Pts',(-1.77606001340043,-0.969474639293403,
-2.18562457894241));
#364519=CARTESIAN_POINT('Ctrl Pts',(-1.9665886161183,-0.476795144252666,
-2.2459421237894));
#364520=CARTESIAN_POINT('Ctrl Pts',(-2.0231790616074,0.0484698229690482,
-2.30639998925771));
#364521=CARTESIAN_POINT('Ctrl Pts',(-1.94138573006516,0.570342005097921,
-2.36685494461854));
#364522=CARTESIAN_POINT('Ctrl Pts',(-1.72773301625381,1.05344259449438,
-2.42717237256682));
#364523=CARTESIAN_POINT('Ctrl Pts',(-1.39633042998923,1.46487729238585,
-2.48762977035772));
#364524=CARTESIAN_POINT('Ctrl Pts',(-0.969474291036093,1.77605966206198,
-2.54808497616048));
#364525=CARTESIAN_POINT('Ctrl Pts',(-0.476795343347378,1.96658811640277,
-2.6084023881129));
#364526=CARTESIAN_POINT('Ctrl Pts',(0.0484699602192744,2.02317939996145,
-2.66885975673847));
#364527=CARTESIAN_POINT('Ctrl Pts',(0.570341982836039,1.94138567238666,
-2.72931497821885));
#364528=CARTESIAN_POINT('Ctrl Pts',(1.05344257210098,1.72773301387229,-2.78963238875962));
#364529=CARTESIAN_POINT('Ctrl Pts',(1.46487731147791,1.39633043581364,-2.85008975616076));
#364530=CARTESIAN_POINT('Ctrl Pts',(1.7760596572503,0.96947429019414,-2.91054497830833));
#364531=CARTESIAN_POINT('Ctrl Pts',(1.96658811657123,0.47679534386094,-2.97086238877306));
#364532=CARTESIAN_POINT('Ctrl Pts',(2.02317940049204,-0.0484699606166185,
-3.03131975614836));
#364533=CARTESIAN_POINT('Ctrl Pts',(1.94138567221384,-0.570341982644115,
-3.09177497831011));
#364534=CARTESIAN_POINT('Ctrl Pts',(1.72773301391076,-1.05344257214956,
-3.15209238877301));
#364535=CARTESIAN_POINT('Ctrl Pts',(1.39633043580907,-1.46487731147983,
-3.21254975614839));
#364536=CARTESIAN_POINT('Ctrl Pts',(0.969474290197969,-1.77605965724421,
-3.27300497831004));
#364537=CARTESIAN_POINT('Ctrl Pts',(0.476795343858464,-1.96658811657341,
-3.33332238877311));
#364538=CARTESIAN_POINT('Ctrl Pts',(-0.0484699606159255,-2.0231794004916,
-3.39377975614832));
#364539=CARTESIAN_POINT('Ctrl Pts',(-0.570341982644268,-1.94138567221424,
-3.45423497831005));
#364540=CARTESIAN_POINT('Ctrl Pts',(-1.05344257214943,-1.72773301391041,
-3.51455238877311));
#364541=CARTESIAN_POINT('Ctrl Pts',(-1.46487731147993,-1.39633043580919,
-3.57500975614831));
#364542=CARTESIAN_POINT('Ctrl Pts',(-1.77605965724425,-0.969474290197954,
-3.63546497831004));
#364543=CARTESIAN_POINT('Ctrl Pts',(-1.96658811657337,-0.476795343858458,
-3.69578238877312));
#364544=CARTESIAN_POINT('Ctrl Pts',(-2.02317940049162,0.0484699606159343,
-3.75623975614831));
#364545=CARTESIAN_POINT('Ctrl Pts',(-1.94138567221425,0.570341982644281,
-3.81669497831005));
#364546=CARTESIAN_POINT('Ctrl Pts',(-1.7277330139104,1.05344257214943,-3.87701238877311));
#364547=CARTESIAN_POINT('Ctrl Pts',(-1.39633043580919,1.46487731147993,
-3.93746975614831));
#364548=CARTESIAN_POINT('Ctrl Pts',(-0.969474290197942,1.77605965724426,
-3.99792497831004));
#364549=CARTESIAN_POINT('Ctrl Pts',(-0.476795343858452,1.96658811657335,
-4.05824238877313));
#364550=CARTESIAN_POINT('Ctrl Pts',(0.0484699606159434,2.02317940049163,
-4.11869975614831));
#364551=CARTESIAN_POINT('Ctrl Pts',(0.570341982644284,1.94138567221424,
-4.17915497831005));
#364552=CARTESIAN_POINT('Ctrl Pts',(1.05344257214943,1.72773301391039,-4.23947238877311));
#364553=CARTESIAN_POINT('Ctrl Pts',(1.46487731147993,1.39633043580918,-4.29992975614832));
#364554=CARTESIAN_POINT('Ctrl Pts',(1.77605965724427,0.969474290197945,
-4.36038497831003));
#364555=CARTESIAN_POINT('Ctrl Pts',(1.96658811657337,0.476795343858441,
-4.42070238877312));
#364556=CARTESIAN_POINT('Ctrl Pts',(2.02317940049162,-0.0484699606159445,
-4.48115975614831));
#364557=CARTESIAN_POINT('Ctrl Pts',(1.94138567221424,-0.570341982644292,
-4.54161497831005));
#364558=CARTESIAN_POINT('Ctrl Pts',(1.72773301391038,-1.05344257214943,
-4.60193238877312));
#364559=CARTESIAN_POINT('Ctrl Pts',(1.39633043580918,-1.46487731147994,
-4.66238975614831));
#364560=CARTESIAN_POINT('Ctrl Pts',(0.969474290197935,-1.77605965724426,
-4.72284497831004));
#364561=CARTESIAN_POINT('Ctrl Pts',(0.476795343858439,-1.96658811657337,
-4.78316238877312));
#364562=CARTESIAN_POINT('Ctrl Pts',(-0.0484699606159579,-2.02317940049164,
-4.8436197561483));
#364563=CARTESIAN_POINT('Ctrl Pts',(-0.570341982644288,-1.94138567221422,
-4.90407497831006));
#364564=CARTESIAN_POINT('Ctrl Pts',(-1.05344257214943,-1.72773301391037,
-4.96439238877312));
#364565=CARTESIAN_POINT('Ctrl Pts',(-1.46487731147995,-1.39633043580918,
-5.02484975614831));
#364566=CARTESIAN_POINT('Ctrl Pts',(-1.77605965724426,-0.969474290197928,
-5.08530497831004));
#364567=CARTESIAN_POINT('Ctrl Pts',(-1.96658811657335,-0.476795343858433,
-5.14562238877313));
#364568=CARTESIAN_POINT('Ctrl Pts',(-2.02317940049163,0.0484699606159606,
-5.2060797561483));
#364569=CARTESIAN_POINT('Ctrl Pts',(-1.94138567221425,0.570341982644311,
-5.26653497831003));
#364570=CARTESIAN_POINT('Ctrl Pts',(-1.72773301391036,1.05344257214944,
-5.32685238877313));
#364571=CARTESIAN_POINT('Ctrl Pts',(-1.39633043580918,1.46487731147996,
-5.3873097561483));
#364572=CARTESIAN_POINT('Ctrl Pts',(-0.969474290197916,1.77605965724424,
-5.44776497831006));
#364573=CARTESIAN_POINT('Ctrl Pts',(-0.476795343858422,1.96658811657339,
-5.5080823887731));
#364574=CARTESIAN_POINT('Ctrl Pts',(0.0484699606159706,2.02317940049163,
-5.56853975614829));
#364575=CARTESIAN_POINT('Ctrl Pts',(0.570341982644291,1.94138567221422,
-5.62899497831007));
#364576=CARTESIAN_POINT('Ctrl Pts',(1.05344257214944,1.72773301391032,-5.68931238877313));
#364577=CARTESIAN_POINT('Ctrl Pts',(1.46487731147996,1.3963304358092,-5.74976975614823));
#364578=CARTESIAN_POINT('Ctrl Pts',(1.77605965724441,0.969474290197947,
-5.81022497831013));
#364579=CARTESIAN_POINT('Ctrl Pts',(1.96658811657315,0.476795343858267,
-5.87054238877304));
#364580=CARTESIAN_POINT('Ctrl Pts',(2.02317940049197,-0.0484699606151168,
-5.93099975614826));
#364581=CARTESIAN_POINT('Ctrl Pts',(1.94138567221262,-0.570341982647331,
-5.99145497831012));
#364582=CARTESIAN_POINT('Ctrl Pts',(1.72773301391079,-1.05344257214282,
-6.05177238877488));
#364583=CARTESIAN_POINT('Ctrl Pts',(1.39633043583791,-1.46487731150212,
-6.1122297561358));
#364584=CARTESIAN_POINT('Ctrl Pts',(0.969474290103704,-1.77605965719443,
-6.17268497832268));
#364585=CARTESIAN_POINT('Ctrl Pts',(0.476795344014053,-1.96658811647506,
-6.23300238886911));
#364586=CARTESIAN_POINT('Ctrl Pts',(-0.0484699607888847,-2.02317940162764,
-6.293459755551));
#364587=CARTESIAN_POINT('Ctrl Pts',(-0.570341982515374,-1.94138566986718,
-6.35391497894857));
#364588=CARTESIAN_POINT('Ctrl Pts',(-1.0534425689941,-1.72773301427299,
-6.41423239105532));
#364589=CARTESIAN_POINT('Ctrl Pts',(-1.46487733129139,-1.39633044764682,
-6.47468974174144));
#364590=CARTESIAN_POINT('Ctrl Pts',(-1.77605962440754,-0.969474272408487,
-6.53514499410053));
#364591=CARTESIAN_POINT('Ctrl Pts',(-1.96658808441403,-0.4767953693466,
-6.59546242507117));
#364592=CARTESIAN_POINT('Ctrl Pts',(-2.02317971788315,0.0484700612956726,
-6.65591951867769));
#364593=CARTESIAN_POINT('Ctrl Pts',(-1.94138529374751,0.57034175258804,
-6.71637524065362));
#364594=CARTESIAN_POINT('Ctrl Pts',(-1.7277327906675,1.05344225923825,-6.77669281345839));
#364595=CARTESIAN_POINT('Ctrl Pts',(-1.39633190064527,1.46488023063332,
-6.83714685373563));
#364596=CARTESIAN_POINT('Ctrl Pts',(-0.969474795144666,1.77605674551469,
-6.89760831895014));
#364597=CARTESIAN_POINT('Ctrl Pts',(-0.476792483974202,1.96658170561334,
-6.95792512927773));
#364598=CARTESIAN_POINT('Ctrl Pts',(0.0484734593030573,2.0232081210323,
-7.01835708981697));
#364599=CARTESIAN_POINT('Ctrl Pts',(0.570336624689882,1.94136175768686,
-7.07885725203471));
#364600=CARTESIAN_POINT('Ctrl Pts',(1.05340619968671,1.72778052727257,-7.13918044053492));
#364601=CARTESIAN_POINT('Ctrl Pts',(1.46503146071072,1.39600002911185,-7.19942807213429));
#364602=CARTESIAN_POINT('Ctrl Pts',(1.77572739170825,0.970967789756964,
-7.26046972816476));
#364603=CARTESIAN_POINT('Ctrl Pts',(1.9679960876878,0.471734127632586,-7.31921124624962));
#364604=CARTESIAN_POINT('Ctrl Pts',(2.00016367750205,0.139563645186354,
-7.36277016686196));
#364605=CARTESIAN_POINT('Ctrl Pts',(2.00016367750204,-0.0349606549172864,
-7.37954989315336));
#364606=CARTESIAN_POINT('',(2.00005141137773,-0.0349509159166537,-1.58027907189674));
#364607=CARTESIAN_POINT('',(1.7237531792885,-0.0252784459846846,-1.66884860356395));
#364608=CARTESIAN_POINT('Origin',(2.00000000329361,-4.46994898412652E-6,
-1.90027906926653));
#364609=CARTESIAN_POINT('',(1.99994859520949,0.0349419760186854,-2.22027906663631));
#364610=CARTESIAN_POINT('Origin',(2.00000000329361,-4.46994898412652E-6,
-1.90027906926653));
#364611=CARTESIAN_POINT('Ctrl Pts',(1.99994859520949,0.0349419760186854,
-2.22027906663631));
#364612=CARTESIAN_POINT('Ctrl Pts',(1.99994859520949,-0.133161143166691,
-2.23644142527053));
#364613=CARTESIAN_POINT('Ctrl Pts',(1.96833139354662,-0.472425718114294,
-2.28062587414611));
#364614=CARTESIAN_POINT('Ctrl Pts',(1.77549751488388,-0.970378153502274,
-2.33932132964638));
#364615=CARTESIAN_POINT('Ctrl Pts',(1.46486827473653,-1.39599810161593,
-2.40041168228136));
#364616=CARTESIAN_POINT('Ctrl Pts',(1.0532724675317,-1.72756949816,-2.46064650153962));
#364617=CARTESIAN_POINT('Ctrl Pts',(0.570253827701872,-1.94116844962337,
-2.52097328730337));
#364618=CARTESIAN_POINT('Ctrl Pts',(0.0484505622703552,-2.02298787581022,
-2.58147196284819));
#364619=CARTESIAN_POINT('Ctrl Pts',(-0.476762817249676,-1.96636546213765,
-2.64190473727344));
#364620=CARTESIAN_POINT('Ctrl Pts',(-0.969389646094711,-1.7758542783469,
-2.70222141276452));
#364621=CARTESIAN_POINT('Ctrl Pts',(-1.39619412835269,-1.46471035101601,
-2.76268238970025));
#364622=CARTESIAN_POINT('Ctrl Pts',(-1.72755848446788,-1.05330968911041,
-2.8231370123091));
#364623=CARTESIAN_POINT('Ctrl Pts',(-1.94118200928605,-0.570259037663673,
-2.88345449584336));
#364624=CARTESIAN_POINT('Ctrl Pts',(-2.02296215046454,-0.0484473116516587,
-2.94390972032538));
#364625=CARTESIAN_POINT('Ctrl Pts',(-1.96637109382515,0.476765855935366,
-3.00436740295728));
#364626=CARTESIAN_POINT('Ctrl Pts',(-1.77585739520295,0.969389009874219,
-3.06468474103924));
#364627=CARTESIAN_POINT('Ctrl Pts',(-1.46470740175196,1.39619269138418,
-3.12513949735647));
#364628=CARTESIAN_POINT('Ctrl Pts',(-1.05331000180424,1.72755870986409,
-3.18559743702838));
#364629=CARTESIAN_POINT('Ctrl Pts',(-0.570259275444307,1.94118238224882,
-3.2459147561141));
#364630=CARTESIAN_POINT('Ctrl Pts',(-0.0484472107178668,2.02296183497224,
-3.30636948355066));
#364631=CARTESIAN_POINT('Ctrl Pts',(0.476765831354286,1.96637112545875,
-3.36682743921798));
#364632=CARTESIAN_POINT('Ctrl Pts',(0.969389026744113,1.77585742843582,
-3.42714475673536));
#364633=CARTESIAN_POINT('Ctrl Pts',(1.39619267971627,1.46470738191116,-3.48759948296635));
#364634=CARTESIAN_POINT('Ctrl Pts',(1.72755870948907,1.05331000492523,-3.54805743931225));
#364635=CARTESIAN_POINT('Ctrl Pts',(1.9411823845861,0.570259275622033,-3.60837475674778));
#364636=CARTESIAN_POINT('Ctrl Pts',(2.02296183383815,0.0484472105365179,
-3.66882948295392));
#364637=CARTESIAN_POINT('Ctrl Pts',(1.96637112555601,-0.476765831198158,
-3.72928743931407));
#364638=CARTESIAN_POINT('Ctrl Pts',(1.77585742848668,-0.969389026837108,
-3.78960475674772));
#364639=CARTESIAN_POINT('Ctrl Pts',(1.46470738188885,-1.39619267968778,
-3.85005948295395));
#364640=CARTESIAN_POINT('Ctrl Pts',(1.05331000493188,-1.72755870948857,
-3.910517439314));
#364641=CARTESIAN_POINT('Ctrl Pts',(0.570259275619007,-1.9411823845877,
-3.97083475674782));
#364642=CARTESIAN_POINT('Ctrl Pts',(0.0484472105373659,-2.02296183383781,
-4.03128948295388));
#364643=CARTESIAN_POINT('Ctrl Pts',(-0.476765831198311,-1.96637112555626,
-4.09174743931402));
#364644=CARTESIAN_POINT('Ctrl Pts',(-0.969389026837092,-1.77585742848654,
-4.15206475674782));
#364645=CARTESIAN_POINT('Ctrl Pts',(-1.39619267968775,-1.46470738188883,
-4.21251948295388));
#364646=CARTESIAN_POINT('Ctrl Pts',(-1.72755870948862,-1.05331000493188,
-4.27297743931401));
#364647=CARTESIAN_POINT('Ctrl Pts',(-1.94118238458768,-0.570259275619005,
-4.33329475674783));
#364648=CARTESIAN_POINT('Ctrl Pts',(-2.0229618338378,-0.0484472105373586,
-4.39374948295387));
#364649=CARTESIAN_POINT('Ctrl Pts',(-1.96637112555625,0.476765831198322,
-4.45420743931402));
#364650=CARTESIAN_POINT('Ctrl Pts',(-1.77585742848654,0.969389026837096,
-4.51452475674782));
#364651=CARTESIAN_POINT('Ctrl Pts',(-1.46470738188882,1.39619267968775,
-4.57497948295388));
#364652=CARTESIAN_POINT('Ctrl Pts',(-1.05331000493187,1.72755870948862,
-4.63543743931401));
#364653=CARTESIAN_POINT('Ctrl Pts',(-0.570259275619004,1.9411823845877,
-4.69575475674784));
#364654=CARTESIAN_POINT('Ctrl Pts',(-0.0484472105373471,2.0229618338378,
-4.75620948295387));
#364655=CARTESIAN_POINT('Ctrl Pts',(0.476765831198326,1.96637112555626,
-4.81666743931402));
#364656=CARTESIAN_POINT('Ctrl Pts',(0.969389026837101,1.77585742848653,
-4.87698475674782));
#364657=CARTESIAN_POINT('Ctrl Pts',(1.39619267968776,1.46470738188882,-4.93743948295388));
#364658=CARTESIAN_POINT('Ctrl Pts',(1.72755870948861,1.05331000493185,-4.997897439314));
#364659=CARTESIAN_POINT('Ctrl Pts',(1.94118238458768,0.570259275618993,
-5.05821475674782));
#364660=CARTESIAN_POINT('Ctrl Pts',(2.0229618338378,0.0484472105373451,
-5.11866948295387));
#364661=CARTESIAN_POINT('Ctrl Pts',(1.96637112555625,-0.476765831198331,
-5.17912743931402));
#364662=CARTESIAN_POINT('Ctrl Pts',(1.77585742848654,-0.969389026837107,
-5.23944475674783));
#364663=CARTESIAN_POINT('Ctrl Pts',(1.46470738188881,-1.39619267968776,
-5.29989948295387));
#364664=CARTESIAN_POINT('Ctrl Pts',(1.05331000493185,-1.72755870948862,
-5.36035743931401));
#364665=CARTESIAN_POINT('Ctrl Pts',(0.57025927561899,-1.94118238458768,
-5.42067475674783));
#364666=CARTESIAN_POINT('Ctrl Pts',(0.0484472105373359,-2.02296183383778,
-5.48112948295386));
#364667=CARTESIAN_POINT('Ctrl Pts',(-0.476765831198329,-1.96637112555626,
-5.54158743931402));
#364668=CARTESIAN_POINT('Ctrl Pts',(-0.96938902683712,-1.77585742848655,
-5.60190475674783));
#364669=CARTESIAN_POINT('Ctrl Pts',(-1.39619267968776,-1.4647073818888,
-5.66235948295387));
#364670=CARTESIAN_POINT('Ctrl Pts',(-1.72755870948862,-1.05331000493185,
-5.722817439314));
#364671=CARTESIAN_POINT('Ctrl Pts',(-1.9411823845877,-0.570259275618991,
-5.78313475674784));
#364672=CARTESIAN_POINT('Ctrl Pts',(-2.02296183383779,-0.0484472105373294,
-5.84358948295386));
#364673=CARTESIAN_POINT('Ctrl Pts',(-1.96637112555623,0.476765831198343,
-5.904047439314));
#364674=CARTESIAN_POINT('Ctrl Pts',(-1.77585742848654,0.969389026837124,
-5.96436475674784));
#364675=CARTESIAN_POINT('Ctrl Pts',(-1.46470738188879,1.39619267968775,
-6.02481948295386));
#364676=CARTESIAN_POINT('Ctrl Pts',(-1.05331000493186,1.72755870948864,
-6.08527743931403));
#364677=CARTESIAN_POINT('Ctrl Pts',(-0.57025927561896,1.94118238458767,
-6.14559475674781));
#364678=CARTESIAN_POINT('Ctrl Pts',(-0.0484472105373227,2.02296183383776,
-6.20604948295386));
#364679=CARTESIAN_POINT('Ctrl Pts',(0.476765831198343,1.96637112555631,
-6.26650743931404));
#364680=CARTESIAN_POINT('Ctrl Pts',(0.969389026837138,1.77585742848649,
-6.32682475674784));
#364681=CARTESIAN_POINT('Ctrl Pts',(1.39619267968763,1.4647073818887,-6.3872794829538));
#364682=CARTESIAN_POINT('Ctrl Pts',(1.72755870948896,1.05331000493196,-6.4477374393141));
#364683=CARTESIAN_POINT('Ctrl Pts',(1.94118238458724,0.570259275618813,
-6.50805475674775));
#364684=CARTESIAN_POINT('Ctrl Pts',(2.0229618338382,0.0484472105380158,
-6.56850948295382));
#364685=CARTESIAN_POINT('Ctrl Pts',(1.96637112555413,-0.47676583120083,
-6.62896743931409));
#364686=CARTESIAN_POINT('Ctrl Pts',(1.77585742849251,-0.969389026833344,
-6.68928475674954));
#364687=CARTESIAN_POINT('Ctrl Pts',(1.46470738188697,-1.39619267969199,
-6.74973948294137));
#364688=CARTESIAN_POINT('Ctrl Pts',(1.05331000488233,-1.72755870945149,
-6.81019743932769));
#364689=CARTESIAN_POINT('Ctrl Pts',(0.570259275809968,-1.94118238475938,
-6.87051475683913));
#364690=CARTESIAN_POINT('Ctrl Pts',(0.0484472101488399,-2.02296183330866,
-6.93096948236246));
#364691=CARTESIAN_POINT('Ctrl Pts',(-0.476765830732716,-1.96637112538019,
-6.99142743997978));
#364692=CARTESIAN_POINT('Ctrl Pts',(-0.969389027651612,-1.775857433288,
-7.05174475889683));
#364693=CARTESIAN_POINT('Ctrl Pts',(-1.39619267380615,-1.46470736293583,
-7.11219946872276));
#364694=CARTESIAN_POINT('Ctrl Pts',(-1.72755871231312,-1.05331002647757,
-7.1726574556236));
#364695=CARTESIAN_POINT('Ctrl Pts',(-1.94118244199894,-0.570259298778077,
-7.23297479041701));
#364696=CARTESIAN_POINT('Ctrl Pts',(-2.02296149561613,-0.0484470734163606,
-7.29342924947211));
#364697=CARTESIAN_POINT('Ctrl Pts',(-1.96637162260829,0.47676563992917,
-7.35388770608518));
#364698=CARTESIAN_POINT('Ctrl Pts',(-1.77585778550465,0.969389377563547,
-7.41420515419699));
#364699=CARTESIAN_POINT('Ctrl Pts',(-1.46470321414872,1.39619055347437,
-7.4746566054593));
#364700=CARTESIAN_POINT('Ctrl Pts',(-1.05331679189158,1.72756279918536,
-7.53512091909894));
#364701=CARTESIAN_POINT('Ctrl Pts',(-0.570256351317271,1.94118541096824,
-7.5954368568002));
#364702=CARTESIAN_POINT('Ctrl Pts',(-0.0484373346474795,2.02291433148142,
-7.65586848775589));
#364703=CARTESIAN_POINT('Ctrl Pts',(0.476753357889169,1.96647633924905,
-7.7163654145941));
#364704=CARTESIAN_POINT('Ctrl Pts',(0.969439733353148,1.77572407380791,
-7.7767079034587));
#364705=CARTESIAN_POINT('Ctrl Pts',(1.39587962475789,1.46484458461224,-7.83687735653918));
#364706=CARTESIAN_POINT('Ctrl Pts',(1.72854436163452,1.05253719801599,-7.89821617217114));
#364707=CARTESIAN_POINT('Ctrl Pts',(1.93848294702123,0.574209674581668,
-7.95584767975511));
#364708=CARTESIAN_POINT('Ctrl Pts',(1.99983638908382,0.21585245779268,-8.0021551741418));
#364709=CARTESIAN_POINT('Ctrl Pts',(1.99983638908381,0.0349322317806574,
-8.0195498399348));
#364710=CARTESIAN_POINT('Ctrl Pts',(2.00005141137773,-0.0349509159166537,
-1.58027907189674));
#364711=CARTESIAN_POINT('Ctrl Pts',(2.00005141137773,-0.209477500702,-1.59705901785001));
#364712=CARTESIAN_POINT('Ctrl Pts',(1.93937485936534,-0.574981221086946,
-1.64398167301615));
#364713=CARTESIAN_POINT('Ctrl Pts',(1.72866575619624,-1.05218683017129,
-1.70157781695483));
#364714=CARTESIAN_POINT('Ctrl Pts',(1.39603065320521,-1.46514475575449,
-1.76296158741006));
#364715=CARTESIAN_POINT('Ctrl Pts',(0.969522180315677,-1.77589106055163,
-1.82311912419573));
#364716=CARTESIAN_POINT('Ctrl Pts',(0.476783238604109,-1.96670288995313,
-1.88346520364747));
#364717=CARTESIAN_POINT('Ctrl Pts',(-0.0484603850821368,-2.02312932285366,
-1.94396055370022));
#364718=CARTESIAN_POINT('Ctrl Pts',(-0.570338856925993,-1.94138942628423,
-2.00439291407465));
#364719=CARTESIAN_POINT('Ctrl Pts',(-1.05344948325284,-1.72773686772633,
-2.06470891120488));
#364720=CARTESIAN_POINT('Ctrl Pts',(-1.46487312544728,-1.39632835696345,
-2.1251726344757));
#364721=CARTESIAN_POINT('Ctrl Pts',(-1.77606001340043,-0.969474639293403,
-2.18562457894241));
#364722=CARTESIAN_POINT('Ctrl Pts',(-1.9665886161183,-0.476795144252666,
-2.2459421237894));
#364723=CARTESIAN_POINT('Ctrl Pts',(-2.0231790616074,0.0484698229690482,
-2.30639998925771));
#364724=CARTESIAN_POINT('Ctrl Pts',(-1.94138573006516,0.570342005097921,
-2.36685494461854));
#364725=CARTESIAN_POINT('Ctrl Pts',(-1.72773301625381,1.05344259449438,
-2.42717237256682));
#364726=CARTESIAN_POINT('Ctrl Pts',(-1.39633042998923,1.46487729238585,
-2.48762977035772));
#364727=CARTESIAN_POINT('Ctrl Pts',(-0.969474291036093,1.77605966206198,
-2.54808497616048));
#364728=CARTESIAN_POINT('Ctrl Pts',(-0.476795343347378,1.96658811640277,
-2.6084023881129));
#364729=CARTESIAN_POINT('Ctrl Pts',(0.0484699602192744,2.02317939996145,
-2.66885975673847));
#364730=CARTESIAN_POINT('Ctrl Pts',(0.570341982836039,1.94138567238666,
-2.72931497821885));
#364731=CARTESIAN_POINT('Ctrl Pts',(1.05344257210098,1.72773301387229,-2.78963238875962));
#364732=CARTESIAN_POINT('Ctrl Pts',(1.46487731147791,1.39633043581364,-2.85008975616076));
#364733=CARTESIAN_POINT('Ctrl Pts',(1.7760596572503,0.96947429019414,-2.91054497830833));
#364734=CARTESIAN_POINT('Ctrl Pts',(1.96658811657123,0.47679534386094,-2.97086238877306));
#364735=CARTESIAN_POINT('Ctrl Pts',(2.02317940049204,-0.0484699606166185,
-3.03131975614836));
#364736=CARTESIAN_POINT('Ctrl Pts',(1.94138567221384,-0.570341982644115,
-3.09177497831011));
#364737=CARTESIAN_POINT('Ctrl Pts',(1.72773301391076,-1.05344257214956,
-3.15209238877301));
#364738=CARTESIAN_POINT('Ctrl Pts',(1.39633043580907,-1.46487731147983,
-3.21254975614839));
#364739=CARTESIAN_POINT('Ctrl Pts',(0.969474290197968,-1.77605965724421,
-3.27300497831004));
#364740=CARTESIAN_POINT('Ctrl Pts',(0.476795343858464,-1.96658811657341,
-3.33332238877311));
#364741=CARTESIAN_POINT('Ctrl Pts',(-0.0484699606159255,-2.0231794004916,
-3.39377975614832));
#364742=CARTESIAN_POINT('Ctrl Pts',(-0.570341982644268,-1.94138567221424,
-3.45423497831005));
#364743=CARTESIAN_POINT('Ctrl Pts',(-1.05344257214943,-1.72773301391041,
-3.51455238877311));
#364744=CARTESIAN_POINT('Ctrl Pts',(-1.46487731147993,-1.39633043580919,
-3.57500975614831));
#364745=CARTESIAN_POINT('Ctrl Pts',(-1.77605965724425,-0.969474290197954,
-3.63546497831004));
#364746=CARTESIAN_POINT('Ctrl Pts',(-1.96658811657337,-0.476795343858458,
-3.69578238877312));
#364747=CARTESIAN_POINT('Ctrl Pts',(-2.02317940049162,0.0484699606159343,
-3.75623975614831));
#364748=CARTESIAN_POINT('Ctrl Pts',(-1.94138567221425,0.570341982644281,
-3.81669497831005));
#364749=CARTESIAN_POINT('Ctrl Pts',(-1.7277330139104,1.05344257214943,-3.87701238877311));
#364750=CARTESIAN_POINT('Ctrl Pts',(-1.39633043580919,1.46487731147993,
-3.93746975614831));
#364751=CARTESIAN_POINT('Ctrl Pts',(-0.969474290197942,1.77605965724426,
-3.99792497831004));
#364752=CARTESIAN_POINT('Ctrl Pts',(-0.476795343858452,1.96658811657335,
-4.05824238877313));
#364753=CARTESIAN_POINT('Ctrl Pts',(0.0484699606159434,2.02317940049163,
-4.11869975614831));
#364754=CARTESIAN_POINT('Ctrl Pts',(0.570341982644284,1.94138567221424,
-4.17915497831005));
#364755=CARTESIAN_POINT('Ctrl Pts',(1.05344257214943,1.72773301391039,-4.23947238877311));
#364756=CARTESIAN_POINT('Ctrl Pts',(1.46487731147993,1.39633043580918,-4.29992975614832));
#364757=CARTESIAN_POINT('Ctrl Pts',(1.77605965724427,0.969474290197945,
-4.36038497831003));
#364758=CARTESIAN_POINT('Ctrl Pts',(1.96658811657337,0.476795343858441,
-4.42070238877312));
#364759=CARTESIAN_POINT('Ctrl Pts',(2.02317940049162,-0.0484699606159445,
-4.48115975614831));
#364760=CARTESIAN_POINT('Ctrl Pts',(1.94138567221424,-0.570341982644292,
-4.54161497831005));
#364761=CARTESIAN_POINT('Ctrl Pts',(1.72773301391038,-1.05344257214943,
-4.60193238877312));
#364762=CARTESIAN_POINT('Ctrl Pts',(1.39633043580918,-1.46487731147994,
-4.66238975614831));
#364763=CARTESIAN_POINT('Ctrl Pts',(0.969474290197935,-1.77605965724426,
-4.72284497831004));
#364764=CARTESIAN_POINT('Ctrl Pts',(0.476795343858439,-1.96658811657337,
-4.78316238877312));
#364765=CARTESIAN_POINT('Ctrl Pts',(-0.0484699606159579,-2.02317940049164,
-4.8436197561483));
#364766=CARTESIAN_POINT('Ctrl Pts',(-0.570341982644288,-1.94138567221422,
-4.90407497831006));
#364767=CARTESIAN_POINT('Ctrl Pts',(-1.05344257214943,-1.72773301391037,
-4.96439238877312));
#364768=CARTESIAN_POINT('Ctrl Pts',(-1.46487731147995,-1.39633043580918,
-5.02484975614831));
#364769=CARTESIAN_POINT('Ctrl Pts',(-1.77605965724426,-0.969474290197928,
-5.08530497831004));
#364770=CARTESIAN_POINT('Ctrl Pts',(-1.96658811657335,-0.476795343858433,
-5.14562238877313));
#364771=CARTESIAN_POINT('Ctrl Pts',(-2.02317940049163,0.0484699606159606,
-5.2060797561483));
#364772=CARTESIAN_POINT('Ctrl Pts',(-1.94138567221425,0.570341982644311,
-5.26653497831003));
#364773=CARTESIAN_POINT('Ctrl Pts',(-1.72773301391036,1.05344257214944,
-5.32685238877313));
#364774=CARTESIAN_POINT('Ctrl Pts',(-1.39633043580918,1.46487731147996,
-5.3873097561483));
#364775=CARTESIAN_POINT('Ctrl Pts',(-0.969474290197916,1.77605965724424,
-5.44776497831006));
#364776=CARTESIAN_POINT('Ctrl Pts',(-0.476795343858422,1.96658811657339,
-5.5080823887731));
#364777=CARTESIAN_POINT('Ctrl Pts',(0.0484699606159706,2.02317940049163,
-5.56853975614829));
#364778=CARTESIAN_POINT('Ctrl Pts',(0.570341982644291,1.94138567221422,
-5.62899497831007));
#364779=CARTESIAN_POINT('Ctrl Pts',(1.05344257214944,1.72773301391032,-5.68931238877313));
#364780=CARTESIAN_POINT('Ctrl Pts',(1.46487731147996,1.3963304358092,-5.74976975614823));
#364781=CARTESIAN_POINT('Ctrl Pts',(1.77605965724441,0.969474290197947,
-5.81022497831013));
#364782=CARTESIAN_POINT('Ctrl Pts',(1.96658811657315,0.476795343858267,
-5.87054238877304));
#364783=CARTESIAN_POINT('Ctrl Pts',(2.02317940049197,-0.0484699606151168,
-5.93099975614826));
#364784=CARTESIAN_POINT('Ctrl Pts',(1.94138567221262,-0.570341982647331,
-5.99145497831012));
#364785=CARTESIAN_POINT('Ctrl Pts',(1.72773301391079,-1.05344257214282,
-6.05177238877488));
#364786=CARTESIAN_POINT('Ctrl Pts',(1.39633043583791,-1.46487731150212,
-6.1122297561358));
#364787=CARTESIAN_POINT('Ctrl Pts',(0.969474290103703,-1.77605965719442,
-6.17268497832268));
#364788=CARTESIAN_POINT('Ctrl Pts',(0.476795344014053,-1.96658811647506,
-6.23300238886911));
#364789=CARTESIAN_POINT('Ctrl Pts',(-0.0484699607888847,-2.02317940162764,
-6.293459755551));
#364790=CARTESIAN_POINT('Ctrl Pts',(-0.570341982515374,-1.94138566986718,
-6.35391497894857));
#364791=CARTESIAN_POINT('Ctrl Pts',(-1.0534425689941,-1.72773301427299,
-6.41423239105532));
#364792=CARTESIAN_POINT('Ctrl Pts',(-1.46487733129139,-1.39633044764682,
-6.47468974174144));
#364793=CARTESIAN_POINT('Ctrl Pts',(-1.77605962440754,-0.969474272408487,
-6.53514499410053));
#364794=CARTESIAN_POINT('Ctrl Pts',(-1.96658808441403,-0.4767953693466,
-6.59546242507117));
#364795=CARTESIAN_POINT('Ctrl Pts',(-2.02317971788315,0.0484700612956726,
-6.65591951867769));
#364796=CARTESIAN_POINT('Ctrl Pts',(-1.94138529374751,0.57034175258804,
-6.71637524065362));
#364797=CARTESIAN_POINT('Ctrl Pts',(-1.7277327906675,1.05344225923825,-6.77669281345839));
#364798=CARTESIAN_POINT('Ctrl Pts',(-1.39633190064527,1.46488023063332,
-6.83714685373563));
#364799=CARTESIAN_POINT('Ctrl Pts',(-0.969474795144666,1.77605674551469,
-6.89760831895014));
#364800=CARTESIAN_POINT('Ctrl Pts',(-0.476792483974202,1.96658170561334,
-6.95792512927773));
#364801=CARTESIAN_POINT('Ctrl Pts',(0.0484734593030573,2.0232081210323,
-7.01835708981697));
#364802=CARTESIAN_POINT('Ctrl Pts',(0.570336624689882,1.94136175768686,
-7.07885725203471));
#364803=CARTESIAN_POINT('Ctrl Pts',(1.05340619968671,1.72778052727257,-7.13918044053492));
#364804=CARTESIAN_POINT('Ctrl Pts',(1.46503146071072,1.39600002911185,-7.19942807213429));
#364805=CARTESIAN_POINT('Ctrl Pts',(1.77572739170825,0.970967789756964,
-7.26046972816476));
#364806=CARTESIAN_POINT('Ctrl Pts',(1.9679960876878,0.471734127632586,-7.31921124624962));
#364807=CARTESIAN_POINT('Ctrl Pts',(2.00016367750205,0.139563645186354,
-7.36277016686196));
#364808=CARTESIAN_POINT('Ctrl Pts',(2.00016367750204,-0.0349606549172864,
-7.37954989315336));
#364809=CARTESIAN_POINT('Ctrl Pts',(2.,0.,-0.919999999999993));
#364810=CARTESIAN_POINT('Ctrl Pts',(1.9924061401935,-0.1305836429736,-0.926868907781472));
#364811=CARTESIAN_POINT('Ctrl Pts',(1.97718154739341,-0.392384998448425,
-0.940640076412341));
#364812=CARTESIAN_POINT('Ctrl Pts',(1.85901893075151,-0.770264472745852,
-0.961199190461979));
#364813=CARTESIAN_POINT('Ctrl Pts',(1.67380212461465,-1.11839049672256,
-0.981867932445977));
#364814=CARTESIAN_POINT('Ctrl Pts',(1.39568858766182,-1.45707298411786,
-1.00483530662099));
#364815=CARTESIAN_POINT('Ctrl Pts',(1.01136330582357,-1.75174676674517,
-1.03005611602139));
#364816=CARTESIAN_POINT('Ctrl Pts',(0.523585702942253,-1.95400607364428,
-1.05751009591307));
#364817=CARTESIAN_POINT('Ctrl Pts',(-1.62435722739463E-5,-2.02307699179836,
-1.08507117314344));
#364818=CARTESIAN_POINT('Ctrl Pts',(-0.523536317885363,-1.95385305544458,
-1.11259298299813));
#364819=CARTESIAN_POINT('Ctrl Pts',(-1.01143313765049,-1.75187888421358,
-1.14006309809451));
#364820=CARTESIAN_POINT('Ctrl Pts',(-1.43055439145378,-1.43053532023484,
-1.16760081034308));
#364821=CARTESIAN_POINT('Ctrl Pts',(-1.7517838724523,-1.01138424804627,
-1.19513433615883));
#364822=CARTESIAN_POINT('Ctrl Pts',(-1.95395118967044,-0.52357502362932,
-1.22260450625386));
#364823=CARTESIAN_POINT('Ctrl Pts',(-2.02309840874517,1.39140831439291E-5,
-1.25013947035447));
#364824=CARTESIAN_POINT('Ctrl Pts',(-1.95385456936267,0.52354165019408,
-1.27767463061609));
#364825=CARTESIAN_POINT('Ctrl Pts',(-1.75187530264009,1.01142844098439,
-1.30514480045556));
#364826=CARTESIAN_POINT('Ctrl Pts',(-1.43053726663428,1.4305573555692,-1.33267812946709));
#364827=CARTESIAN_POINT('Ctrl Pts',(-1.01138541561949,1.75178358667915,
-1.36021604426028));
#364828=CARTESIAN_POINT('Ctrl Pts',(-0.523570999948669,1.95394672745918,
-1.38768613982889));
#364829=CARTESIAN_POINT('Ctrl Pts',(1.24423377236111E-5,2.02310883807685,
-1.41520780852107));
#364830=CARTESIAN_POINT('Ctrl Pts',(0.523542096174336,1.95385181633148,
-1.44276890960603));
#364831=CARTESIAN_POINT('Ctrl Pts',(1.0114195685531,1.75192189566403,-1.47022354238125));
#364832=CARTESIAN_POINT('Ctrl Pts',(1.39574727856968,1.45690129136922,-1.49544185654267));
#364833=CARTESIAN_POINT('Ctrl Pts',(1.67373453408061,1.11891073119414,-1.51841614397666));
#364834=CARTESIAN_POINT('Ctrl Pts',(1.85897590932335,0.768114988005871,
-1.53906122201719));
#364835=CARTESIAN_POINT('Ctrl Pts',(1.97776901413901,0.398755552237307,
-1.55979576815126));
#364836=CARTESIAN_POINT('Ctrl Pts',(1.99260464990788,0.109993480400852,
-1.57343356620573));
#364837=CARTESIAN_POINT('Ctrl Pts',(2.00005141137773,-0.0349509159166537,
-1.58027907189674));
#364838=CARTESIAN_POINT('Ctrl Pts',(2.8,0.,-0.919999999999993));
#364839=CARTESIAN_POINT('Ctrl Pts',(2.78939199277986,-0.182993728026944,
-0.926864406801388));
#364840=CARTESIAN_POINT('Ctrl Pts',(2.76812446948309,-0.54986973906403,
-0.940626551616868));
#364841=CARTESIAN_POINT('Ctrl Pts',(2.60295543055419,-1.07729524714901,
-0.961278164543689));
#364842=CARTESIAN_POINT('Ctrl Pts',(2.3432740748819,-1.56601868287461,-0.981972834586931));
#364843=CARTESIAN_POINT('Ctrl Pts',(1.9534645938062,-2.04021452969416,-1.00482284429261));
#364844=CARTESIAN_POINT('Ctrl Pts',(1.41694431361456,-2.45199325498274,
-1.02999729271682));
#364845=CARTESIAN_POINT('Ctrl Pts',(0.732261973497512,-2.73592828705718,
-1.05766533228683));
#364846=CARTESIAN_POINT('Ctrl Pts',(-5.53107937837186E-5,-2.83213060052566,
-1.08508982617781));
#364847=CARTESIAN_POINT('Ctrl Pts',(-0.732227236330921,-2.73573484730789,
-1.11255527546237));
#364848=CARTESIAN_POINT('Ctrl Pts',(-1.41671668511953,-2.4523342703758,
-1.14018764997613));
#364849=CARTESIAN_POINT('Ctrl Pts',(-2.00264985801735,-2.00263363186375,
-1.16763896370469));
#364850=CARTESIAN_POINT('Ctrl Pts',(-2.4522378702943,-1.41666694884076,
-1.19509582612308));
#364851=CARTESIAN_POINT('Ctrl Pts',(-2.73582334389193,-0.732298418914319,
-1.22272542915656));
#364852=CARTESIAN_POINT('Ctrl Pts',(-2.83216647994848,1.05873370328634E-5,
-1.25018040117675));
#364853=CARTESIAN_POINT('Ctrl Pts',(-2.73572815948738,0.732260080199856,
-1.27763556928937));
#364854=CARTESIAN_POINT('Ctrl Pts',(-2.4523317981686,1.41670660974565,-1.30526517206592));
#364855=CARTESIAN_POINT('Ctrl Pts',(-2.0026374388973,2.0026509689249,-1.33272183775651));
#364856=CARTESIAN_POINT('Ctrl Pts',(-1.41667347271186,2.45223646417305,
-1.3601733539516));
#364857=CARTESIAN_POINT('Ctrl Pts',(-0.73226691430792,2.73582715423785,
-1.38780570894782));
#364858=CARTESIAN_POINT('Ctrl Pts',(-3.32541419378344E-5,2.83216215152901,
-1.41527101711875));
#364859=CARTESIAN_POINT('Ctrl Pts',(0.732213474069494,2.73577655753039,
-1.44269553505523));
#364860=CARTESIAN_POINT('Ctrl Pts',(1.41699596320263,2.45216677851596,-1.47036422641732));
#364861=CARTESIAN_POINT('Ctrl Pts',(1.95351849625047,2.04006124129144,-1.49553618329511));
#364862=CARTESIAN_POINT('Ctrl Pts',(2.34320434404536,1.56650518466477,-1.51839309578454));
#364863=CARTESIAN_POINT('Ctrl Pts',(2.60290758877066,1.07529461519169,-1.5390641373972));
#364864=CARTESIAN_POINT('Ctrl Pts',(2.7689186260588,0.55507555381449,-1.55989143937075));
#364865=CARTESIAN_POINT('Ctrl Pts',(2.78964685205658,0.162241467065363,
-1.57352004288224));
#364866=CARTESIAN_POINT('Ctrl Pts',(2.80005140479051,-0.0349419760186688,
-1.58036093336367));
#364867=CARTESIAN_POINT('Ctrl Pts',(2.8,0.,-1.55999999999999));
#364868=CARTESIAN_POINT('Ctrl Pts',(2.78939649751634,-0.182997808095028,
-1.56686440711942));
#364869=CARTESIAN_POINT('Ctrl Pts',(2.76813800556597,-0.549881999079696,
-1.58062655257252));
#364870=CARTESIAN_POINT('Ctrl Pts',(2.60287048343998,-1.07724179710562,
-1.6012781606252));
#364871=CARTESIAN_POINT('Ctrl Pts',(2.34315963754124,-1.56595368435367,
-1.62197282719421));
#364872=CARTESIAN_POINT('Ctrl Pts',(1.95348731824777,-2.04021286575323,
-1.64482284638796));
#364873=CARTESIAN_POINT('Ctrl Pts',(1.41697144358507,-2.45206379948272,
-1.66999729490308));
#364874=CARTESIAN_POINT('Ctrl Pts',(0.732200851511023,-2.73574151657536,
-1.69766532043691));
#364875=CARTESIAN_POINT('Ctrl Pts',(-2.70481749242659E-5,-2.83210623547185,
-1.72508982747625));
#364876=CARTESIAN_POINT('Ctrl Pts',(-0.732252487208887,-2.73577889971119,
-1.75255527725563));
#364877=CARTESIAN_POINT('Ctrl Pts',(-1.41664649586044,-2.45219160028545,
-1.78018764150562));
#364878=CARTESIAN_POINT('Ctrl Pts',(-2.00259639972156,-2.00261890380741,
-1.80763896342095));
#364879=CARTESIAN_POINT('Ctrl Pts',(-2.45228673495991,-1.41668180042844,
-1.83509582821663));
#364880=CARTESIAN_POINT('Ctrl Pts',(-2.73567754904204,-0.732247710943258,
-1.86272542106748));
#364881=CARTESIAN_POINT('Ctrl Pts',(-2.83211473644778,-1.68757765071671E-5,
-1.89018040067487));
#364882=CARTESIAN_POINT('Ctrl Pts',(-2.73577394601168,0.732284104217307,
-1.91763557143196));
#364883=CARTESIAN_POINT('Ctrl Pts',(-2.45219333916896,1.41663986613312,
-1.94526516399832));
#364884=CARTESIAN_POINT('Ctrl Pts',(-2.00261772079364,2.00259272042701,
-1.9727218371175));
#364885=CARTESIAN_POINT('Ctrl Pts',(-1.41669182241623,2.4522887952019,-2.00017335617694));
#364886=CARTESIAN_POINT('Ctrl Pts',(-0.732214969721451,2.73568587053461,
-2.02780570068256));
#364887=CARTESIAN_POINT('Ctrl Pts',(-6.15112143014144E-5,2.83207265142351,
-2.05527101556769));
#364888=CARTESIAN_POINT('Ctrl Pts',(0.732247904310314,2.73590203116,-2.08269553782593));
#364889=CARTESIAN_POINT('Ctrl Pts',(1.41691695808072,2.45186224921218,-2.11036421584428));
#364890=CARTESIAN_POINT('Ctrl Pts',(1.95342442139249,2.04047105442842,-2.13553617856065));
#364891=CARTESIAN_POINT('Ctrl Pts',(2.34323316729515,1.56520434188013,-2.15839309657528));
#364892=CARTESIAN_POINT('Ctrl Pts',(2.60289731690865,1.08024771508786,-2.17906413834116));
#364893=CARTESIAN_POINT('Ctrl Pts',(2.76880371833477,0.536476428508159,
-2.19989143334533));
#364894=CARTESIAN_POINT('Ctrl Pts',(2.7895399948989,0.202560389138996,-2.21352003736615));
#364895=CARTESIAN_POINT('Ctrl Pts',(2.79994858862227,0.0349509159166703,
-2.22036092810323));
#364896=CARTESIAN_POINT('Ctrl Pts',(2.,0.,-1.55999999999999));
#364897=CARTESIAN_POINT('Ctrl Pts',(1.99241064492998,-0.130587723041684,
-1.56686890809951));
#364898=CARTESIAN_POINT('Ctrl Pts',(1.97719508347629,-0.392397258464091,
-1.58064007736799));
#364899=CARTESIAN_POINT('Ctrl Pts',(1.85893398363731,-0.77021102270246,
-1.60119918654349));
#364900=CARTESIAN_POINT('Ctrl Pts',(1.67368768727399,-1.11832549820161,
-1.62186792505326));
#364901=CARTESIAN_POINT('Ctrl Pts',(1.39571131210339,-1.45707132017693,
-1.64483530871634));
#364902=CARTESIAN_POINT('Ctrl Pts',(1.01139043579407,-1.75181731124514,
-1.67005611820765));
#364903=CARTESIAN_POINT('Ctrl Pts',(0.523524580955764,-1.95381930316246,
-1.69751008406315));
#364904=CARTESIAN_POINT('Ctrl Pts',(1.20190465855827E-5,-2.02305262674455,
-1.72507117444189));
#364905=CARTESIAN_POINT('Ctrl Pts',(-0.523561568763329,-1.95389710784788,
-1.75259298479139));
#364906=CARTESIAN_POINT('Ctrl Pts',(-1.0113629483914,-1.75173621412323,
-1.780063089624));
#364907=CARTESIAN_POINT('Ctrl Pts',(-1.43050093315799,-1.4305205921785,
-1.80760081005934));
#364908=CARTESIAN_POINT('Ctrl Pts',(-1.75183273711791,-1.01139909963394,
-1.83513433825238));
#364909=CARTESIAN_POINT('Ctrl Pts',(-1.95380539482055,-0.523524315658259,
-1.86260449816478));
#364910=CARTESIAN_POINT('Ctrl Pts',(-2.02304666524447,-1.35490303961885E-5,
-1.89013946985259));
#364911=CARTESIAN_POINT('Ctrl Pts',(-1.95390035588696,0.523565674211531,
-1.91767463275868));
#364912=CARTESIAN_POINT('Ctrl Pts',(-1.75173684364045,1.01136169737186,
-1.94514479238796));
#364913=CARTESIAN_POINT('Ctrl Pts',(-1.43051754853062,1.43049910707131,
-1.97267812882809));
#364914=CARTESIAN_POINT('Ctrl Pts',(-1.01140376532386,1.751835917708,-2.00021604648563));
#364915=CARTESIAN_POINT('Ctrl Pts',(-0.523519055362199,1.95380544375593,
-2.02768613156363));
#364916=CARTESIAN_POINT('Ctrl Pts',(-1.58147346400669E-5,2.02301933797135,
-2.05520780697));
#364917=CARTESIAN_POINT('Ctrl Pts',(0.523576526415156,1.95397728996109,
-2.08276891237674));
#364918=CARTESIAN_POINT('Ctrl Pts',(1.01134056343118,1.75161736636026,-2.11022353180821));
#364919=CARTESIAN_POINT('Ctrl Pts',(1.3956532037117,1.4573111045062,-2.13544185180822));
#364920=CARTESIAN_POINT('Ctrl Pts',(1.67376335733039,1.1176098884095,-2.1584161447674));
#364921=CARTESIAN_POINT('Ctrl Pts',(1.85896563746134,0.773068087902041,
-2.17906122296115));
#364922=CARTESIAN_POINT('Ctrl Pts',(1.97765410641497,0.380156426930975,
-2.19979576212585));
#364923=CARTESIAN_POINT('Ctrl Pts',(1.9924977927502,0.150312402474485,-2.21343356068965));
#364924=CARTESIAN_POINT('Ctrl Pts',(1.99994859520949,0.0349419760186854,
-2.22027906663631));
#364925=CARTESIAN_POINT('Ctrl Pts',(1.2,0.,-1.55999999999999));
#364926=CARTESIAN_POINT('Ctrl Pts',(1.19542479234362,-0.0781776379883396,
-1.56687340907959));
#364927=CARTESIAN_POINT('Ctrl Pts',(1.18625216138661,-0.234912517848486,
-1.58065360216347));
#364928=CARTESIAN_POINT('Ctrl Pts',(1.11499748383463,-0.4631802482993,-1.60112021246178));
#364929=CARTESIAN_POINT('Ctrl Pts',(1.00421573700674,-0.670697312049558,
-1.62176302291231));
#364930=CARTESIAN_POINT('Ctrl Pts',(0.837935305959016,-0.873929774600632,
-1.64484777104472));
#364931=CARTESIAN_POINT('Ctrl Pts',(0.60580942800308,-1.05157082300757,
-1.67011494151222));
#364932=CARTESIAN_POINT('Ctrl Pts',(0.314848310400505,-1.17189708974956,
-1.6973548476894));
#364933=CARTESIAN_POINT('Ctrl Pts',(5.10862680953333E-5,-1.21399901801725,
-1.72505252140752));
#364934=CARTESIAN_POINT('Ctrl Pts',(-0.31487065031777,-1.17201531598458,
-1.75263069232715));
#364935=CARTESIAN_POINT('Ctrl Pts',(-0.606079400922359,-1.05128082796102,
-1.77993853774237));
#364936=CARTESIAN_POINT('Ctrl Pts',(-0.858405466594417,-0.858422280549586,
-1.80756265669772));
#364937=CARTESIAN_POINT('Ctrl Pts',(-1.0513787392759,-0.606116398839451,
-1.83517284828813));
#364938=CARTESIAN_POINT('Ctrl Pts',(-1.17193324059906,-0.31480092037326,
-1.86248357526207));
#364939=CARTESIAN_POINT('Ctrl Pts',(-1.21397859404116,-1.02222842850628E-5,
-1.89009853903031));
#364940=CARTESIAN_POINT('Ctrl Pts',(-1.17202676576225,0.314847244205754,
-1.9177136940854));
#364941=CARTESIAN_POINT('Ctrl Pts',(-1.05128034811194,0.606083528610609,
-1.9450244207776));
#364942=CARTESIAN_POINT('Ctrl Pts',(-0.858417376267602,0.858405493715605,
-1.97263442053868));
#364943=CARTESIAN_POINT('Ctrl Pts',(-0.606115708231486,1.05138304021409,
-2.00025873679431));
#364944=CARTESIAN_POINT('Ctrl Pts',(-0.314823141002948,1.17192501697726,
-2.0275665624447));
#364945=CARTESIAN_POINT('Ctrl Pts',(2.98817450213404E-5,1.21396602451919,
-2.05514459837232));
#364946=CARTESIAN_POINT('Ctrl Pts',(0.314905148519997,1.17205254876217,
-2.08284228692754));
#364947=CARTESIAN_POINT('Ctrl Pts',(0.605764168781643,1.05137248350833,
-2.11008284777213));
#364948=CARTESIAN_POINT('Ctrl Pts',(0.837881986030918,0.874151154583981,
-2.13534752505579));
#364949=CARTESIAN_POINT('Ctrl Pts',(1.00429354736563,0.670015434938871,
-2.15843919295953));
#364950=CARTESIAN_POINT('Ctrl Pts',(1.11503395801403,0.465888460716222,
-2.17905830758114));
#364951=CARTESIAN_POINT('Ctrl Pts',(1.18650449449518,0.223836425353792,
-2.19970009090637));
#364952=CARTESIAN_POINT('Ctrl Pts',(1.1954555906015,0.0980644158099734,
-2.21334708401314));
#364953=CARTESIAN_POINT('Ctrl Pts',(1.19994860179671,0.0349330361207006,
-2.22019720516939));
#364954=CARTESIAN_POINT('Ctrl Pts',(1.2,0.,-0.919999999999993));
#364955=CARTESIAN_POINT('Ctrl Pts',(1.19542028760714,-0.0781735579202564,
-0.926873408761556));
#364956=CARTESIAN_POINT('Ctrl Pts',(1.18623862530372,-0.23490025783282,
-0.940653601207814));
#364957=CARTESIAN_POINT('Ctrl Pts',(1.11508243094883,-0.463233698342691,
-0.961120216380269));
#364958=CARTESIAN_POINT('Ctrl Pts',(1.0043301743474,-0.670762310570501,
-0.981763030305022));
#364959=CARTESIAN_POINT('Ctrl Pts',(0.837912581517445,-0.873931438541563,
-1.00484776894937));
#364960=CARTESIAN_POINT('Ctrl Pts',(0.605782298032579,-1.0515002785076,
-1.03011493932597));
#364961=CARTESIAN_POINT('Ctrl Pts',(0.314909432386994,-1.17208386023138,
-1.05735485953932));
#364962=CARTESIAN_POINT('Ctrl Pts',(2.28236492357989E-5,-1.21402338307106,
-1.08505252010907));
#364963=CARTESIAN_POINT('Ctrl Pts',(-0.314845399439805,-1.17197126358128,
-1.11263069053389));
#364964=CARTESIAN_POINT('Ctrl Pts',(-0.606149590181453,-1.05142349805137,
-1.13993854621288));
#364965=CARTESIAN_POINT('Ctrl Pts',(-0.858458924890206,-0.858437008605928,
-1.16756265698147));
#364966=CARTESIAN_POINT('Ctrl Pts',(-1.05132987461029,-0.606101547251777,
-1.19517284619458));
#364967=CARTESIAN_POINT('Ctrl Pts',(-1.17207903544895,-0.314851628344321,
-1.22248358335115));
#364968=CARTESIAN_POINT('Ctrl Pts',(-1.21403033754186,1.72408292549676E-5,
-1.25009853953219));
#364969=CARTESIAN_POINT('Ctrl Pts',(-1.17198097923795,0.314823220188304,
-1.27771369194281));
#364970=CARTESIAN_POINT('Ctrl Pts',(-1.05141880711158,0.60615027222314,
-1.3050244288452));
#364971=CARTESIAN_POINT('Ctrl Pts',(-0.858437094371262,0.858463742213499,
-1.33263442117768));
#364972=CARTESIAN_POINT('Ctrl Pts',(-0.606097358527115,1.05133070918524,
-1.36025873456897));
#364973=CARTESIAN_POINT('Ctrl Pts',(-0.314875085589417,1.1720663006805,
-1.38756657070996));
#364974=CARTESIAN_POINT('Ctrl Pts',(5.81388173850348E-5,1.21405552462469,
-1.41514459992339));
#364975=CARTESIAN_POINT('Ctrl Pts',(0.314870718279177,1.17192707513256,
-1.44284228415683));
#364976=CARTESIAN_POINT('Ctrl Pts',(0.60584317390356,1.05167701281211,-1.47008285834517));
#364977=CARTESIAN_POINT('Ctrl Pts',(0.837976060888895,0.873741341447001,
-1.49534752979024));
#364978=CARTESIAN_POINT('Ctrl Pts',(1.00426472411585,0.671316277723509,
-1.51843919216879));
#364979=CARTESIAN_POINT('Ctrl Pts',(1.11504422987604,0.460935360820052,
-1.53905830663718));
#364980=CARTESIAN_POINT('Ctrl Pts',(1.18661940221922,0.242435550660123,
-1.55970009693178));
#364981=CARTESIAN_POINT('Ctrl Pts',(1.19556244775918,0.0577454937363405,
-1.57334708952923));
#364982=CARTESIAN_POINT('Ctrl Pts',(1.20005141796495,-0.0349598558146385,
-1.58019721042982));
#364983=CARTESIAN_POINT('Ctrl Pts',(2.,0.,-0.919999999999993));
#364984=CARTESIAN_POINT('Ctrl Pts',(1.9924061401935,-0.1305836429736,-0.926868907781472));
#364985=CARTESIAN_POINT('Ctrl Pts',(1.97718154739341,-0.392384998448425,
-0.940640076412341));
#364986=CARTESIAN_POINT('Ctrl Pts',(1.85901893075151,-0.770264472745852,
-0.961199190461979));
#364987=CARTESIAN_POINT('Ctrl Pts',(1.67380212461465,-1.11839049672256,
-0.981867932445977));
#364988=CARTESIAN_POINT('Ctrl Pts',(1.39568858766182,-1.45707298411786,
-1.00483530662099));
#364989=CARTESIAN_POINT('Ctrl Pts',(1.01136330582357,-1.75174676674517,
-1.03005611602139));
#364990=CARTESIAN_POINT('Ctrl Pts',(0.523585702942253,-1.95400607364428,
-1.05751009591307));
#364991=CARTESIAN_POINT('Ctrl Pts',(-1.62435722739463E-5,-2.02307699179836,
-1.08507117314344));
#364992=CARTESIAN_POINT('Ctrl Pts',(-0.523536317885363,-1.95385305544458,
-1.11259298299813));
#364993=CARTESIAN_POINT('Ctrl Pts',(-1.01143313765049,-1.75187888421358,
-1.14006309809451));
#364994=CARTESIAN_POINT('Ctrl Pts',(-1.43055439145378,-1.43053532023484,
-1.16760081034308));
#364995=CARTESIAN_POINT('Ctrl Pts',(-1.7517838724523,-1.01138424804627,
-1.19513433615883));
#364996=CARTESIAN_POINT('Ctrl Pts',(-1.95395118967044,-0.52357502362932,
-1.22260450625386));
#364997=CARTESIAN_POINT('Ctrl Pts',(-2.02309840874517,1.39140831439291E-5,
-1.25013947035447));
#364998=CARTESIAN_POINT('Ctrl Pts',(-1.95385456936267,0.52354165019408,
-1.27767463061609));
#364999=CARTESIAN_POINT('Ctrl Pts',(-1.75187530264009,1.01142844098439,
-1.30514480045556));
#365000=CARTESIAN_POINT('Ctrl Pts',(-1.43053726663428,1.4305573555692,-1.33267812946709));
#365001=CARTESIAN_POINT('Ctrl Pts',(-1.01138541561949,1.75178358667915,
-1.36021604426028));
#365002=CARTESIAN_POINT('Ctrl Pts',(-0.523570999948669,1.95394672745918,
-1.38768613982889));
#365003=CARTESIAN_POINT('Ctrl Pts',(1.24423377236111E-5,2.02310883807685,
-1.41520780852107));
#365004=CARTESIAN_POINT('Ctrl Pts',(0.523542096174336,1.95385181633148,
-1.44276890960603));
#365005=CARTESIAN_POINT('Ctrl Pts',(1.0114195685531,1.75192189566403,-1.47022354238125));
#365006=CARTESIAN_POINT('Ctrl Pts',(1.39574727856968,1.45690129136922,-1.49544185654267));
#365007=CARTESIAN_POINT('Ctrl Pts',(1.67373453408061,1.11891073119414,-1.51841614397666));
#365008=CARTESIAN_POINT('Ctrl Pts',(1.85897590932335,0.768114988005871,
-1.53906122201719));
#365009=CARTESIAN_POINT('Ctrl Pts',(1.97776901413901,0.398755552237307,
-1.55979576815126));
#365010=CARTESIAN_POINT('Ctrl Pts',(1.99260464990788,0.109993480400852,
-1.57343356620573));
#365011=CARTESIAN_POINT('Ctrl Pts',(2.00005141137773,-0.0349509159166537,
-1.58027907189674));
#365012=CARTESIAN_POINT('',(2.,0.,-1.55999999999999));
#365013=CARTESIAN_POINT('',(2.,0.,-0.919999999999993));
#365014=CARTESIAN_POINT('Origin',(2.,0.,-1.23999999999999));
#365015=CARTESIAN_POINT('Ctrl Pts',(2.,0.,-1.55999999999999));
#365016=CARTESIAN_POINT('Ctrl Pts',(1.99241064492998,-0.130587723041684,
-1.56686890809951));
#365017=CARTESIAN_POINT('Ctrl Pts',(1.97719508347629,-0.392397258464091,
-1.58064007736799));
#365018=CARTESIAN_POINT('Ctrl Pts',(1.85893398363731,-0.77021102270246,
-1.60119918654349));
#365019=CARTESIAN_POINT('Ctrl Pts',(1.67368768727399,-1.11832549820161,
-1.62186792505326));
#365020=CARTESIAN_POINT('Ctrl Pts',(1.39571131210339,-1.45707132017693,
-1.64483530871634));
#365021=CARTESIAN_POINT('Ctrl Pts',(1.01139043579407,-1.75181731124514,
-1.67005611820765));
#365022=CARTESIAN_POINT('Ctrl Pts',(0.523524580955764,-1.95381930316246,
-1.69751008406315));
#365023=CARTESIAN_POINT('Ctrl Pts',(1.20190465855827E-5,-2.02305262674455,
-1.72507117444189));
#365024=CARTESIAN_POINT('Ctrl Pts',(-0.523561568763329,-1.95389710784788,
-1.75259298479139));
#365025=CARTESIAN_POINT('Ctrl Pts',(-1.0113629483914,-1.75173621412323,
-1.780063089624));
#365026=CARTESIAN_POINT('Ctrl Pts',(-1.43050093315799,-1.4305205921785,
-1.80760081005934));
#365027=CARTESIAN_POINT('Ctrl Pts',(-1.75183273711791,-1.01139909963394,
-1.83513433825238));
#365028=CARTESIAN_POINT('Ctrl Pts',(-1.95380539482055,-0.523524315658259,
-1.86260449816478));
#365029=CARTESIAN_POINT('Ctrl Pts',(-2.02304666524447,-1.35490303961885E-5,
-1.89013946985259));
#365030=CARTESIAN_POINT('Ctrl Pts',(-1.95390035588696,0.523565674211531,
-1.91767463275868));
#365031=CARTESIAN_POINT('Ctrl Pts',(-1.75173684364045,1.01136169737186,
-1.94514479238796));
#365032=CARTESIAN_POINT('Ctrl Pts',(-1.43051754853062,1.43049910707131,
-1.97267812882809));
#365033=CARTESIAN_POINT('Ctrl Pts',(-1.01140376532386,1.751835917708,-2.00021604648563));
#365034=CARTESIAN_POINT('Ctrl Pts',(-0.523519055362199,1.95380544375593,
-2.02768613156363));
#365035=CARTESIAN_POINT('Ctrl Pts',(-1.58147346400669E-5,2.02301933797135,
-2.05520780697));
#365036=CARTESIAN_POINT('Ctrl Pts',(0.523576526415156,1.95397728996109,
-2.08276891237674));
#365037=CARTESIAN_POINT('Ctrl Pts',(1.01134056343118,1.75161736636026,-2.11022353180821));
#365038=CARTESIAN_POINT('Ctrl Pts',(1.3956532037117,1.4573111045062,-2.13544185180822));
#365039=CARTESIAN_POINT('Ctrl Pts',(1.67376335733039,1.1176098884095,-2.1584161447674));
#365040=CARTESIAN_POINT('Ctrl Pts',(1.85896563746134,0.773068087902041,
-2.17906122296115));
#365041=CARTESIAN_POINT('Ctrl Pts',(1.97765410641497,0.380156426930975,
-2.19979576212585));
#365042=CARTESIAN_POINT('Ctrl Pts',(1.9924977927502,0.150312402474485,-2.21343356068965));
#365043=CARTESIAN_POINT('Ctrl Pts',(1.99994859520949,0.0349419760186854,
-2.22027906663631));
#365044=CARTESIAN_POINT('Ctrl Pts',(2.,0.,-0.919999999999993));
#365045=CARTESIAN_POINT('Ctrl Pts',(1.9924061401935,-0.1305836429736,-0.926868907781472));
#365046=CARTESIAN_POINT('Ctrl Pts',(1.97718154739341,-0.392384998448425,
-0.940640076412341));
#365047=CARTESIAN_POINT('Ctrl Pts',(1.85901893075151,-0.770264472745852,
-0.961199190461979));
#365048=CARTESIAN_POINT('Ctrl Pts',(1.67380212461465,-1.11839049672256,
-0.981867932445977));
#365049=CARTESIAN_POINT('Ctrl Pts',(1.39568858766182,-1.45707298411786,
-1.00483530662099));
#365050=CARTESIAN_POINT('Ctrl Pts',(1.01136330582357,-1.75174676674517,
-1.03005611602139));
#365051=CARTESIAN_POINT('Ctrl Pts',(0.523585702942253,-1.95400607364428,
-1.05751009591307));
#365052=CARTESIAN_POINT('Ctrl Pts',(-1.62435722739463E-5,-2.02307699179836,
-1.08507117314344));
#365053=CARTESIAN_POINT('Ctrl Pts',(-0.523536317885363,-1.95385305544458,
-1.11259298299813));
#365054=CARTESIAN_POINT('Ctrl Pts',(-1.01143313765049,-1.75187888421358,
-1.14006309809451));
#365055=CARTESIAN_POINT('Ctrl Pts',(-1.43055439145378,-1.43053532023484,
-1.16760081034308));
#365056=CARTESIAN_POINT('Ctrl Pts',(-1.7517838724523,-1.01138424804627,
-1.19513433615883));
#365057=CARTESIAN_POINT('Ctrl Pts',(-1.95395118967044,-0.52357502362932,
-1.22260450625386));
#365058=CARTESIAN_POINT('Ctrl Pts',(-2.02309840874517,1.39140831439291E-5,
-1.25013947035447));
#365059=CARTESIAN_POINT('Ctrl Pts',(-1.95385456936267,0.52354165019408,
-1.27767463061609));
#365060=CARTESIAN_POINT('Ctrl Pts',(-1.75187530264009,1.01142844098439,
-1.30514480045556));
#365061=CARTESIAN_POINT('Ctrl Pts',(-1.43053726663428,1.4305573555692,-1.33267812946709));
#365062=CARTESIAN_POINT('Ctrl Pts',(-1.01138541561949,1.75178358667915,
-1.36021604426028));
#365063=CARTESIAN_POINT('Ctrl Pts',(-0.523570999948669,1.95394672745918,
-1.38768613982889));
#365064=CARTESIAN_POINT('Ctrl Pts',(1.24423377236111E-5,2.02310883807685,
-1.41520780852107));
#365065=CARTESIAN_POINT('Ctrl Pts',(0.523542096174336,1.95385181633148,
-1.44276890960603));
#365066=CARTESIAN_POINT('Ctrl Pts',(1.0114195685531,1.75192189566403,-1.47022354238125));
#365067=CARTESIAN_POINT('Ctrl Pts',(1.39574727856968,1.45690129136922,-1.49544185654267));
#365068=CARTESIAN_POINT('Ctrl Pts',(1.67373453408061,1.11891073119414,-1.51841614397666));
#365069=CARTESIAN_POINT('Ctrl Pts',(1.85897590932335,0.768114988005871,
-1.53906122201719));
#365070=CARTESIAN_POINT('Ctrl Pts',(1.97776901413901,0.398755552237307,
-1.55979576815126));
#365071=CARTESIAN_POINT('Ctrl Pts',(1.99260464990788,0.109993480400852,
-1.57343356620573));
#365072=CARTESIAN_POINT('Ctrl Pts',(2.00005141137773,-0.0349509159166537,
-1.58027907189674));
#365073=CARTESIAN_POINT('Ctrl Pts',(2.,0.,-0.919999999999993));
#365074=CARTESIAN_POINT('Ctrl Pts',(1.9924061401935,-0.1305836429736,-0.926868907781472));
#365075=CARTESIAN_POINT('Ctrl Pts',(1.97718154739341,-0.392384998448425,
-0.940640076412341));
#365076=CARTESIAN_POINT('Ctrl Pts',(1.85901893075151,-0.770264472745852,
-0.961199190461979));
#365077=CARTESIAN_POINT('Ctrl Pts',(1.67380212461465,-1.11839049672256,
-0.981867932445977));
#365078=CARTESIAN_POINT('Ctrl Pts',(1.39568858766182,-1.45707298411786,
-1.00483530662099));
#365079=CARTESIAN_POINT('Ctrl Pts',(1.01136330582357,-1.75174676674517,
-1.03005611602139));
#365080=CARTESIAN_POINT('Ctrl Pts',(0.523585702942253,-1.95400607364428,
-1.05751009591307));
#365081=CARTESIAN_POINT('Ctrl Pts',(-1.62435722739463E-5,-2.02307699179836,
-1.08507117314344));
#365082=CARTESIAN_POINT('Ctrl Pts',(-0.523536317885363,-1.95385305544458,
-1.11259298299813));
#365083=CARTESIAN_POINT('Ctrl Pts',(-1.01143313765049,-1.75187888421358,
-1.14006309809451));
#365084=CARTESIAN_POINT('Ctrl Pts',(-1.43055439145378,-1.43053532023484,
-1.16760081034308));
#365085=CARTESIAN_POINT('Ctrl Pts',(-1.7517838724523,-1.01138424804627,
-1.19513433615883));
#365086=CARTESIAN_POINT('Ctrl Pts',(-1.95395118967044,-0.52357502362932,
-1.22260450625386));
#365087=CARTESIAN_POINT('Ctrl Pts',(-2.02309840874517,1.39140831439291E-5,
-1.25013947035447));
#365088=CARTESIAN_POINT('Ctrl Pts',(-1.95385456936267,0.52354165019408,
-1.27767463061609));
#365089=CARTESIAN_POINT('Ctrl Pts',(-1.75187530264009,1.01142844098439,
-1.30514480045556));
#365090=CARTESIAN_POINT('Ctrl Pts',(-1.43053726663428,1.4305573555692,-1.33267812946709));
#365091=CARTESIAN_POINT('Ctrl Pts',(-1.01138541561949,1.75178358667915,
-1.36021604426028));
#365092=CARTESIAN_POINT('Ctrl Pts',(-0.523570999948669,1.95394672745918,
-1.38768613982889));
#365093=CARTESIAN_POINT('Ctrl Pts',(1.24423377236111E-5,2.02310883807685,
-1.41520780852107));
#365094=CARTESIAN_POINT('Ctrl Pts',(0.523542096174336,1.95385181633148,
-1.44276890960603));
#365095=CARTESIAN_POINT('Ctrl Pts',(1.0114195685531,1.75192189566403,-1.47022354238125));
#365096=CARTESIAN_POINT('Ctrl Pts',(1.39574727856968,1.45690129136922,-1.49544185654267));
#365097=CARTESIAN_POINT('Ctrl Pts',(1.67373453408061,1.11891073119414,-1.51841614397666));
#365098=CARTESIAN_POINT('Ctrl Pts',(1.85897590932335,0.768114988005871,
-1.53906122201719));
#365099=CARTESIAN_POINT('Ctrl Pts',(1.97776901413901,0.398755552237307,
-1.55979576815126));
#365100=CARTESIAN_POINT('Ctrl Pts',(1.99260464990788,0.109993480400852,
-1.57343356620573));
#365101=CARTESIAN_POINT('Ctrl Pts',(2.00005141137773,-0.0349509159166537,
-1.58027907189674));
#365102=CARTESIAN_POINT('Ctrl Pts',(2.8,0.,-0.919999999999993));
#365103=CARTESIAN_POINT('Ctrl Pts',(2.78939199277986,-0.182993728026944,
-0.926864406801388));
#365104=CARTESIAN_POINT('Ctrl Pts',(2.76812446948309,-0.54986973906403,
-0.940626551616868));
#365105=CARTESIAN_POINT('Ctrl Pts',(2.60295543055419,-1.07729524714901,
-0.961278164543689));
#365106=CARTESIAN_POINT('Ctrl Pts',(2.3432740748819,-1.56601868287461,-0.981972834586931));
#365107=CARTESIAN_POINT('Ctrl Pts',(1.9534645938062,-2.04021452969416,-1.00482284429261));
#365108=CARTESIAN_POINT('Ctrl Pts',(1.41694431361456,-2.45199325498274,
-1.02999729271682));
#365109=CARTESIAN_POINT('Ctrl Pts',(0.732261973497512,-2.73592828705718,
-1.05766533228683));
#365110=CARTESIAN_POINT('Ctrl Pts',(-5.53107937837186E-5,-2.83213060052566,
-1.08508982617781));
#365111=CARTESIAN_POINT('Ctrl Pts',(-0.732227236330921,-2.73573484730789,
-1.11255527546237));
#365112=CARTESIAN_POINT('Ctrl Pts',(-1.41671668511953,-2.4523342703758,
-1.14018764997613));
#365113=CARTESIAN_POINT('Ctrl Pts',(-2.00264985801735,-2.00263363186375,
-1.16763896370469));
#365114=CARTESIAN_POINT('Ctrl Pts',(-2.4522378702943,-1.41666694884076,
-1.19509582612308));
#365115=CARTESIAN_POINT('Ctrl Pts',(-2.73582334389193,-0.732298418914319,
-1.22272542915656));
#365116=CARTESIAN_POINT('Ctrl Pts',(-2.83216647994848,1.05873370328634E-5,
-1.25018040117675));
#365117=CARTESIAN_POINT('Ctrl Pts',(-2.73572815948738,0.732260080199856,
-1.27763556928937));
#365118=CARTESIAN_POINT('Ctrl Pts',(-2.4523317981686,1.41670660974565,-1.30526517206592));
#365119=CARTESIAN_POINT('Ctrl Pts',(-2.0026374388973,2.0026509689249,-1.33272183775651));
#365120=CARTESIAN_POINT('Ctrl Pts',(-1.41667347271186,2.45223646417305,
-1.3601733539516));
#365121=CARTESIAN_POINT('Ctrl Pts',(-0.73226691430792,2.73582715423785,
-1.38780570894782));
#365122=CARTESIAN_POINT('Ctrl Pts',(-3.32541419378344E-5,2.83216215152901,
-1.41527101711875));
#365123=CARTESIAN_POINT('Ctrl Pts',(0.732213474069494,2.73577655753039,
-1.44269553505523));
#365124=CARTESIAN_POINT('Ctrl Pts',(1.41699596320263,2.45216677851596,-1.47036422641732));
#365125=CARTESIAN_POINT('Ctrl Pts',(1.95351849625047,2.04006124129144,-1.49553618329511));
#365126=CARTESIAN_POINT('Ctrl Pts',(2.34320434404536,1.56650518466477,-1.51839309578454));
#365127=CARTESIAN_POINT('Ctrl Pts',(2.60290758877066,1.07529461519169,-1.5390641373972));
#365128=CARTESIAN_POINT('Ctrl Pts',(2.7689186260588,0.55507555381449,-1.55989143937075));
#365129=CARTESIAN_POINT('Ctrl Pts',(2.78964685205658,0.162241467065363,
-1.57352004288224));
#365130=CARTESIAN_POINT('Ctrl Pts',(2.80005140479051,-0.0349419760186688,
-1.58036093336367));
#365131=CARTESIAN_POINT('Ctrl Pts',(2.8,0.,-1.55999999999999));
#365132=CARTESIAN_POINT('Ctrl Pts',(2.78939649751634,-0.182997808095028,
-1.56686440711942));
#365133=CARTESIAN_POINT('Ctrl Pts',(2.76813800556597,-0.549881999079696,
-1.58062655257252));
#365134=CARTESIAN_POINT('Ctrl Pts',(2.60287048343998,-1.07724179710562,
-1.6012781606252));
#365135=CARTESIAN_POINT('Ctrl Pts',(2.34315963754124,-1.56595368435367,
-1.62197282719421));
#365136=CARTESIAN_POINT('Ctrl Pts',(1.95348731824777,-2.04021286575323,
-1.64482284638796));
#365137=CARTESIAN_POINT('Ctrl Pts',(1.41697144358507,-2.45206379948272,
-1.66999729490308));
#365138=CARTESIAN_POINT('Ctrl Pts',(0.732200851511023,-2.73574151657536,
-1.69766532043691));
#365139=CARTESIAN_POINT('Ctrl Pts',(-2.70481749242659E-5,-2.83210623547185,
-1.72508982747625));
#365140=CARTESIAN_POINT('Ctrl Pts',(-0.732252487208887,-2.73577889971119,
-1.75255527725563));
#365141=CARTESIAN_POINT('Ctrl Pts',(-1.41664649586044,-2.45219160028545,
-1.78018764150562));
#365142=CARTESIAN_POINT('Ctrl Pts',(-2.00259639972156,-2.00261890380741,
-1.80763896342095));
#365143=CARTESIAN_POINT('Ctrl Pts',(-2.45228673495991,-1.41668180042844,
-1.83509582821663));
#365144=CARTESIAN_POINT('Ctrl Pts',(-2.73567754904204,-0.732247710943258,
-1.86272542106748));
#365145=CARTESIAN_POINT('Ctrl Pts',(-2.83211473644778,-1.68757765071671E-5,
-1.89018040067487));
#365146=CARTESIAN_POINT('Ctrl Pts',(-2.73577394601168,0.732284104217307,
-1.91763557143196));
#365147=CARTESIAN_POINT('Ctrl Pts',(-2.45219333916896,1.41663986613312,
-1.94526516399832));
#365148=CARTESIAN_POINT('Ctrl Pts',(-2.00261772079364,2.00259272042701,
-1.9727218371175));
#365149=CARTESIAN_POINT('Ctrl Pts',(-1.41669182241623,2.4522887952019,-2.00017335617694));
#365150=CARTESIAN_POINT('Ctrl Pts',(-0.732214969721451,2.73568587053461,
-2.02780570068256));
#365151=CARTESIAN_POINT('Ctrl Pts',(-6.15112143014144E-5,2.83207265142351,
-2.05527101556769));
#365152=CARTESIAN_POINT('Ctrl Pts',(0.732247904310314,2.73590203116,-2.08269553782593));
#365153=CARTESIAN_POINT('Ctrl Pts',(1.41691695808072,2.45186224921218,-2.11036421584428));
#365154=CARTESIAN_POINT('Ctrl Pts',(1.95342442139249,2.04047105442842,-2.13553617856065));
#365155=CARTESIAN_POINT('Ctrl Pts',(2.34323316729515,1.56520434188013,-2.15839309657528));
#365156=CARTESIAN_POINT('Ctrl Pts',(2.60289731690865,1.08024771508786,-2.17906413834116));
#365157=CARTESIAN_POINT('Ctrl Pts',(2.76880371833477,0.536476428508159,
-2.19989143334533));
#365158=CARTESIAN_POINT('Ctrl Pts',(2.7895399948989,0.202560389138996,-2.21352003736615));
#365159=CARTESIAN_POINT('Ctrl Pts',(2.79994858862227,0.0349509159166703,
-2.22036092810323));
#365160=CARTESIAN_POINT('Ctrl Pts',(2.,0.,-1.55999999999999));
#365161=CARTESIAN_POINT('Ctrl Pts',(1.99241064492998,-0.130587723041684,
-1.56686890809951));
#365162=CARTESIAN_POINT('Ctrl Pts',(1.97719508347629,-0.392397258464091,
-1.58064007736799));
#365163=CARTESIAN_POINT('Ctrl Pts',(1.85893398363731,-0.77021102270246,
-1.60119918654349));
#365164=CARTESIAN_POINT('Ctrl Pts',(1.67368768727399,-1.11832549820161,
-1.62186792505326));
#365165=CARTESIAN_POINT('Ctrl Pts',(1.39571131210339,-1.45707132017693,
-1.64483530871634));
#365166=CARTESIAN_POINT('Ctrl Pts',(1.01139043579407,-1.75181731124514,
-1.67005611820765));
#365167=CARTESIAN_POINT('Ctrl Pts',(0.523524580955764,-1.95381930316246,
-1.69751008406315));
#365168=CARTESIAN_POINT('Ctrl Pts',(1.20190465855827E-5,-2.02305262674455,
-1.72507117444189));
#365169=CARTESIAN_POINT('Ctrl Pts',(-0.523561568763329,-1.95389710784788,
-1.75259298479139));
#365170=CARTESIAN_POINT('Ctrl Pts',(-1.0113629483914,-1.75173621412323,
-1.780063089624));
#365171=CARTESIAN_POINT('Ctrl Pts',(-1.43050093315799,-1.4305205921785,
-1.80760081005934));
#365172=CARTESIAN_POINT('Ctrl Pts',(-1.75183273711791,-1.01139909963394,
-1.83513433825238));
#365173=CARTESIAN_POINT('Ctrl Pts',(-1.95380539482055,-0.523524315658259,
-1.86260449816478));
#365174=CARTESIAN_POINT('Ctrl Pts',(-2.02304666524447,-1.35490303961885E-5,
-1.89013946985259));
#365175=CARTESIAN_POINT('Ctrl Pts',(-1.95390035588696,0.523565674211531,
-1.91767463275868));
#365176=CARTESIAN_POINT('Ctrl Pts',(-1.75173684364045,1.01136169737186,
-1.94514479238796));
#365177=CARTESIAN_POINT('Ctrl Pts',(-1.43051754853062,1.43049910707131,
-1.97267812882809));
#365178=CARTESIAN_POINT('Ctrl Pts',(-1.01140376532386,1.751835917708,-2.00021604648563));
#365179=CARTESIAN_POINT('Ctrl Pts',(-0.523519055362199,1.95380544375593,
-2.02768613156363));
#365180=CARTESIAN_POINT('Ctrl Pts',(-1.58147346400669E-5,2.02301933797135,
-2.05520780697));
#365181=CARTESIAN_POINT('Ctrl Pts',(0.523576526415156,1.95397728996109,
-2.08276891237674));
#365182=CARTESIAN_POINT('Ctrl Pts',(1.01134056343118,1.75161736636026,-2.11022353180821));
#365183=CARTESIAN_POINT('Ctrl Pts',(1.3956532037117,1.4573111045062,-2.13544185180822));
#365184=CARTESIAN_POINT('Ctrl Pts',(1.67376335733039,1.1176098884095,-2.1584161447674));
#365185=CARTESIAN_POINT('Ctrl Pts',(1.85896563746134,0.773068087902041,
-2.17906122296115));
#365186=CARTESIAN_POINT('Ctrl Pts',(1.97765410641497,0.380156426930975,
-2.19979576212585));
#365187=CARTESIAN_POINT('Ctrl Pts',(1.9924977927502,0.150312402474485,-2.21343356068965));
#365188=CARTESIAN_POINT('Ctrl Pts',(1.99994859520949,0.0349419760186854,
-2.22027906663631));
#365189=CARTESIAN_POINT('Ctrl Pts',(1.2,0.,-1.55999999999999));
#365190=CARTESIAN_POINT('Ctrl Pts',(1.19542479234362,-0.0781776379883396,
-1.56687340907959));
#365191=CARTESIAN_POINT('Ctrl Pts',(1.18625216138661,-0.234912517848486,
-1.58065360216347));
#365192=CARTESIAN_POINT('Ctrl Pts',(1.11499748383463,-0.4631802482993,-1.60112021246178));
#365193=CARTESIAN_POINT('Ctrl Pts',(1.00421573700674,-0.670697312049558,
-1.62176302291231));
#365194=CARTESIAN_POINT('Ctrl Pts',(0.837935305959016,-0.873929774600632,
-1.64484777104472));
#365195=CARTESIAN_POINT('Ctrl Pts',(0.60580942800308,-1.05157082300757,
-1.67011494151222));
#365196=CARTESIAN_POINT('Ctrl Pts',(0.314848310400505,-1.17189708974956,
-1.6973548476894));
#365197=CARTESIAN_POINT('Ctrl Pts',(5.10862680953333E-5,-1.21399901801725,
-1.72505252140752));
#365198=CARTESIAN_POINT('Ctrl Pts',(-0.31487065031777,-1.17201531598458,
-1.75263069232715));
#365199=CARTESIAN_POINT('Ctrl Pts',(-0.606079400922359,-1.05128082796102,
-1.77993853774237));
#365200=CARTESIAN_POINT('Ctrl Pts',(-0.858405466594417,-0.858422280549586,
-1.80756265669772));
#365201=CARTESIAN_POINT('Ctrl Pts',(-1.0513787392759,-0.606116398839451,
-1.83517284828813));
#365202=CARTESIAN_POINT('Ctrl Pts',(-1.17193324059906,-0.31480092037326,
-1.86248357526207));
#365203=CARTESIAN_POINT('Ctrl Pts',(-1.21397859404116,-1.02222842850628E-5,
-1.89009853903031));
#365204=CARTESIAN_POINT('Ctrl Pts',(-1.17202676576225,0.314847244205754,
-1.9177136940854));
#365205=CARTESIAN_POINT('Ctrl Pts',(-1.05128034811194,0.606083528610609,
-1.9450244207776));
#365206=CARTESIAN_POINT('Ctrl Pts',(-0.858417376267602,0.858405493715605,
-1.97263442053868));
#365207=CARTESIAN_POINT('Ctrl Pts',(-0.606115708231486,1.05138304021409,
-2.00025873679431));
#365208=CARTESIAN_POINT('Ctrl Pts',(-0.314823141002948,1.17192501697726,
-2.0275665624447));
#365209=CARTESIAN_POINT('Ctrl Pts',(2.98817450213404E-5,1.21396602451919,
-2.05514459837232));
#365210=CARTESIAN_POINT('Ctrl Pts',(0.314905148519997,1.17205254876217,
-2.08284228692754));
#365211=CARTESIAN_POINT('Ctrl Pts',(0.605764168781643,1.05137248350833,
-2.11008284777213));
#365212=CARTESIAN_POINT('Ctrl Pts',(0.837881986030918,0.874151154583981,
-2.13534752505579));
#365213=CARTESIAN_POINT('Ctrl Pts',(1.00429354736563,0.670015434938871,
-2.15843919295953));
#365214=CARTESIAN_POINT('Ctrl Pts',(1.11503395801403,0.465888460716222,
-2.17905830758114));
#365215=CARTESIAN_POINT('Ctrl Pts',(1.18650449449518,0.223836425353792,
-2.19970009090637));
#365216=CARTESIAN_POINT('Ctrl Pts',(1.1954555906015,0.0980644158099734,
-2.21334708401314));
#365217=CARTESIAN_POINT('Ctrl Pts',(1.19994860179671,0.0349330361207006,
-2.22019720516939));
#365218=CARTESIAN_POINT('Ctrl Pts',(1.2,0.,-0.919999999999993));
#365219=CARTESIAN_POINT('Ctrl Pts',(1.19542028760714,-0.0781735579202564,
-0.926873408761556));
#365220=CARTESIAN_POINT('Ctrl Pts',(1.18623862530372,-0.23490025783282,
-0.940653601207814));
#365221=CARTESIAN_POINT('Ctrl Pts',(1.11508243094883,-0.463233698342691,
-0.961120216380269));
#365222=CARTESIAN_POINT('Ctrl Pts',(1.0043301743474,-0.670762310570501,
-0.981763030305022));
#365223=CARTESIAN_POINT('Ctrl Pts',(0.837912581517445,-0.873931438541563,
-1.00484776894937));
#365224=CARTESIAN_POINT('Ctrl Pts',(0.605782298032579,-1.0515002785076,
-1.03011493932597));
#365225=CARTESIAN_POINT('Ctrl Pts',(0.314909432386994,-1.17208386023138,
-1.05735485953932));
#365226=CARTESIAN_POINT('Ctrl Pts',(2.28236492357989E-5,-1.21402338307106,
-1.08505252010907));
#365227=CARTESIAN_POINT('Ctrl Pts',(-0.314845399439805,-1.17197126358128,
-1.11263069053389));
#365228=CARTESIAN_POINT('Ctrl Pts',(-0.606149590181453,-1.05142349805137,
-1.13993854621288));
#365229=CARTESIAN_POINT('Ctrl Pts',(-0.858458924890206,-0.858437008605928,
-1.16756265698147));
#365230=CARTESIAN_POINT('Ctrl Pts',(-1.05132987461029,-0.606101547251777,
-1.19517284619458));
#365231=CARTESIAN_POINT('Ctrl Pts',(-1.17207903544895,-0.314851628344321,
-1.22248358335115));
#365232=CARTESIAN_POINT('Ctrl Pts',(-1.21403033754186,1.72408292549676E-5,
-1.25009853953219));
#365233=CARTESIAN_POINT('Ctrl Pts',(-1.17198097923795,0.314823220188304,
-1.27771369194281));
#365234=CARTESIAN_POINT('Ctrl Pts',(-1.05141880711158,0.60615027222314,
-1.3050244288452));
#365235=CARTESIAN_POINT('Ctrl Pts',(-0.858437094371262,0.858463742213499,
-1.33263442117768));
#365236=CARTESIAN_POINT('Ctrl Pts',(-0.606097358527115,1.05133070918524,
-1.36025873456897));
#365237=CARTESIAN_POINT('Ctrl Pts',(-0.314875085589417,1.1720663006805,
-1.38756657070996));
#365238=CARTESIAN_POINT('Ctrl Pts',(5.81388173850348E-5,1.21405552462469,
-1.41514459992339));
#365239=CARTESIAN_POINT('Ctrl Pts',(0.314870718279177,1.17192707513256,
-1.44284228415683));
#365240=CARTESIAN_POINT('Ctrl Pts',(0.60584317390356,1.05167701281211,-1.47008285834517));
#365241=CARTESIAN_POINT('Ctrl Pts',(0.837976060888895,0.873741341447001,
-1.49534752979024));
#365242=CARTESIAN_POINT('Ctrl Pts',(1.00426472411585,0.671316277723509,
-1.51843919216879));
#365243=CARTESIAN_POINT('Ctrl Pts',(1.11504422987604,0.460935360820052,
-1.53905830663718));
#365244=CARTESIAN_POINT('Ctrl Pts',(1.18661940221922,0.242435550660123,
-1.55970009693178));
#365245=CARTESIAN_POINT('Ctrl Pts',(1.19556244775918,0.0577454937363405,
-1.57334708952923));
#365246=CARTESIAN_POINT('Ctrl Pts',(1.20005141796495,-0.0349598558146385,
-1.58019721042982));
#365247=CARTESIAN_POINT('Ctrl Pts',(2.,0.,-0.919999999999993));
#365248=CARTESIAN_POINT('Ctrl Pts',(1.9924061401935,-0.1305836429736,-0.926868907781472));
#365249=CARTESIAN_POINT('Ctrl Pts',(1.97718154739341,-0.392384998448425,
-0.940640076412341));
#365250=CARTESIAN_POINT('Ctrl Pts',(1.85901893075151,-0.770264472745852,
-0.961199190461979));
#365251=CARTESIAN_POINT('Ctrl Pts',(1.67380212461465,-1.11839049672256,
-0.981867932445977));
#365252=CARTESIAN_POINT('Ctrl Pts',(1.39568858766182,-1.45707298411786,
-1.00483530662099));
#365253=CARTESIAN_POINT('Ctrl Pts',(1.01136330582357,-1.75174676674517,
-1.03005611602139));
#365254=CARTESIAN_POINT('Ctrl Pts',(0.523585702942253,-1.95400607364428,
-1.05751009591307));
#365255=CARTESIAN_POINT('Ctrl Pts',(-1.62435722739463E-5,-2.02307699179836,
-1.08507117314344));
#365256=CARTESIAN_POINT('Ctrl Pts',(-0.523536317885363,-1.95385305544458,
-1.11259298299813));
#365257=CARTESIAN_POINT('Ctrl Pts',(-1.01143313765049,-1.75187888421358,
-1.14006309809451));
#365258=CARTESIAN_POINT('Ctrl Pts',(-1.43055439145378,-1.43053532023484,
-1.16760081034308));
#365259=CARTESIAN_POINT('Ctrl Pts',(-1.7517838724523,-1.01138424804627,
-1.19513433615883));
#365260=CARTESIAN_POINT('Ctrl Pts',(-1.95395118967044,-0.52357502362932,
-1.22260450625386));
#365261=CARTESIAN_POINT('Ctrl Pts',(-2.02309840874517,1.39140831439291E-5,
-1.25013947035447));
#365262=CARTESIAN_POINT('Ctrl Pts',(-1.95385456936267,0.52354165019408,
-1.27767463061609));
#365263=CARTESIAN_POINT('Ctrl Pts',(-1.75187530264009,1.01142844098439,
-1.30514480045556));
#365264=CARTESIAN_POINT('Ctrl Pts',(-1.43053726663428,1.4305573555692,-1.33267812946709));
#365265=CARTESIAN_POINT('Ctrl Pts',(-1.01138541561949,1.75178358667915,
-1.36021604426028));
#365266=CARTESIAN_POINT('Ctrl Pts',(-0.523570999948669,1.95394672745918,
-1.38768613982889));
#365267=CARTESIAN_POINT('Ctrl Pts',(1.24423377236111E-5,2.02310883807685,
-1.41520780852107));
#365268=CARTESIAN_POINT('Ctrl Pts',(0.523542096174336,1.95385181633148,
-1.44276890960603));
#365269=CARTESIAN_POINT('Ctrl Pts',(1.0114195685531,1.75192189566403,-1.47022354238125));
#365270=CARTESIAN_POINT('Ctrl Pts',(1.39574727856968,1.45690129136922,-1.49544185654267));
#365271=CARTESIAN_POINT('Ctrl Pts',(1.67373453408061,1.11891073119414,-1.51841614397666));
#365272=CARTESIAN_POINT('Ctrl Pts',(1.85897590932335,0.768114988005871,
-1.53906122201719));
#365273=CARTESIAN_POINT('Ctrl Pts',(1.97776901413901,0.398755552237307,
-1.55979576815126));
#365274=CARTESIAN_POINT('Ctrl Pts',(1.99260464990788,0.109993480400852,
-1.57343356620573));
#365275=CARTESIAN_POINT('Ctrl Pts',(2.00005141137773,-0.0349509159166537,
-1.58027907189674));
#365276=CARTESIAN_POINT('Origin',(2.,0.,-1.23999999999999));
#365277=CARTESIAN_POINT('',(2.27188945184575,0.0256276272719289,-2.13498880343698));
#365278=CARTESIAN_POINT('Origin',(2.00000000329361,-4.46994898409183E-6,
-1.90027906926653));
#365279=CARTESIAN_POINT('Origin',(2.00000000329361,-4.46994898409183E-6,
-1.90027906926653));
#365280=CARTESIAN_POINT('Origin',(2.,0.,-1.23999999999999));
#365281=CARTESIAN_POINT('Ctrl Pts',(2.00005141137773,-0.0349509159166537,
-1.58027907189674));
#365282=CARTESIAN_POINT('Ctrl Pts',(2.00005141137773,-0.209477500702,-1.59705901785001));
#365283=CARTESIAN_POINT('Ctrl Pts',(1.93937485936534,-0.574981221086946,
-1.64398167301615));
#365284=CARTESIAN_POINT('Ctrl Pts',(1.72866575619624,-1.05218683017129,
-1.70157781695483));
#365285=CARTESIAN_POINT('Ctrl Pts',(1.39603065320521,-1.46514475575449,
-1.76296158741006));
#365286=CARTESIAN_POINT('Ctrl Pts',(0.969522180315677,-1.77589106055163,
-1.82311912419573));
#365287=CARTESIAN_POINT('Ctrl Pts',(0.476783238604109,-1.96670288995313,
-1.88346520364747));
#365288=CARTESIAN_POINT('Ctrl Pts',(-0.0484603850821368,-2.02312932285366,
-1.94396055370022));
#365289=CARTESIAN_POINT('Ctrl Pts',(-0.570338856925993,-1.94138942628423,
-2.00439291407465));
#365290=CARTESIAN_POINT('Ctrl Pts',(-1.05344948325284,-1.72773686772633,
-2.06470891120488));
#365291=CARTESIAN_POINT('Ctrl Pts',(-1.46487312544728,-1.39632835696345,
-2.1251726344757));
#365292=CARTESIAN_POINT('Ctrl Pts',(-1.77606001340043,-0.969474639293403,
-2.18562457894241));
#365293=CARTESIAN_POINT('Ctrl Pts',(-1.9665886161183,-0.476795144252666,
-2.2459421237894));
#365294=CARTESIAN_POINT('Ctrl Pts',(-2.0231790616074,0.0484698229690482,
-2.30639998925771));
#365295=CARTESIAN_POINT('Ctrl Pts',(-1.94138573006516,0.570342005097921,
-2.36685494461854));
#365296=CARTESIAN_POINT('Ctrl Pts',(-1.72773301625381,1.05344259449438,
-2.42717237256682));
#365297=CARTESIAN_POINT('Ctrl Pts',(-1.39633042998923,1.46487729238585,
-2.48762977035772));
#365298=CARTESIAN_POINT('Ctrl Pts',(-0.969474291036093,1.77605966206198,
-2.54808497616048));
#365299=CARTESIAN_POINT('Ctrl Pts',(-0.476795343347378,1.96658811640277,
-2.6084023881129));
#365300=CARTESIAN_POINT('Ctrl Pts',(0.0484699602192744,2.02317939996145,
-2.66885975673847));
#365301=CARTESIAN_POINT('Ctrl Pts',(0.570341982836039,1.94138567238666,
-2.72931497821885));
#365302=CARTESIAN_POINT('Ctrl Pts',(1.05344257210098,1.72773301387229,-2.78963238875962));
#365303=CARTESIAN_POINT('Ctrl Pts',(1.46487731147791,1.39633043581364,-2.85008975616076));
#365304=CARTESIAN_POINT('Ctrl Pts',(1.7760596572503,0.96947429019414,-2.91054497830833));
#365305=CARTESIAN_POINT('Ctrl Pts',(1.96658811657123,0.47679534386094,-2.97086238877306));
#365306=CARTESIAN_POINT('Ctrl Pts',(2.02317940049204,-0.0484699606166185,
-3.03131975614836));
#365307=CARTESIAN_POINT('Ctrl Pts',(1.94138567221384,-0.570341982644115,
-3.09177497831011));
#365308=CARTESIAN_POINT('Ctrl Pts',(1.72773301391076,-1.05344257214956,
-3.15209238877301));
#365309=CARTESIAN_POINT('Ctrl Pts',(1.39633043580907,-1.46487731147983,
-3.21254975614839));
#365310=CARTESIAN_POINT('Ctrl Pts',(0.969474290197969,-1.77605965724421,
-3.27300497831004));
#365311=CARTESIAN_POINT('Ctrl Pts',(0.476795343858464,-1.96658811657341,
-3.33332238877311));
#365312=CARTESIAN_POINT('Ctrl Pts',(-0.0484699606159255,-2.0231794004916,
-3.39377975614832));
#365313=CARTESIAN_POINT('Ctrl Pts',(-0.570341982644268,-1.94138567221424,
-3.45423497831005));
#365314=CARTESIAN_POINT('Ctrl Pts',(-1.05344257214943,-1.72773301391041,
-3.51455238877311));
#365315=CARTESIAN_POINT('Ctrl Pts',(-1.46487731147993,-1.39633043580919,
-3.57500975614831));
#365316=CARTESIAN_POINT('Ctrl Pts',(-1.77605965724425,-0.969474290197954,
-3.63546497831004));
#365317=CARTESIAN_POINT('Ctrl Pts',(-1.96658811657337,-0.476795343858458,
-3.69578238877312));
#365318=CARTESIAN_POINT('Ctrl Pts',(-2.02317940049162,0.0484699606159343,
-3.75623975614831));
#365319=CARTESIAN_POINT('Ctrl Pts',(-1.94138567221425,0.570341982644281,
-3.81669497831005));
#365320=CARTESIAN_POINT('Ctrl Pts',(-1.7277330139104,1.05344257214943,-3.87701238877311));
#365321=CARTESIAN_POINT('Ctrl Pts',(-1.39633043580919,1.46487731147993,
-3.93746975614831));
#365322=CARTESIAN_POINT('Ctrl Pts',(-0.969474290197942,1.77605965724426,
-3.99792497831004));
#365323=CARTESIAN_POINT('Ctrl Pts',(-0.476795343858452,1.96658811657335,
-4.05824238877313));
#365324=CARTESIAN_POINT('Ctrl Pts',(0.0484699606159434,2.02317940049163,
-4.11869975614831));
#365325=CARTESIAN_POINT('Ctrl Pts',(0.570341982644284,1.94138567221424,
-4.17915497831005));
#365326=CARTESIAN_POINT('Ctrl Pts',(1.05344257214943,1.72773301391039,-4.23947238877311));
#365327=CARTESIAN_POINT('Ctrl Pts',(1.46487731147993,1.39633043580918,-4.29992975614832));
#365328=CARTESIAN_POINT('Ctrl Pts',(1.77605965724427,0.969474290197945,
-4.36038497831003));
#365329=CARTESIAN_POINT('Ctrl Pts',(1.96658811657337,0.476795343858441,
-4.42070238877312));
#365330=CARTESIAN_POINT('Ctrl Pts',(2.02317940049162,-0.0484699606159445,
-4.48115975614831));
#365331=CARTESIAN_POINT('Ctrl Pts',(1.94138567221424,-0.570341982644292,
-4.54161497831005));
#365332=CARTESIAN_POINT('Ctrl Pts',(1.72773301391038,-1.05344257214943,
-4.60193238877312));
#365333=CARTESIAN_POINT('Ctrl Pts',(1.39633043580918,-1.46487731147994,
-4.66238975614831));
#365334=CARTESIAN_POINT('Ctrl Pts',(0.969474290197935,-1.77605965724426,
-4.72284497831004));
#365335=CARTESIAN_POINT('Ctrl Pts',(0.476795343858439,-1.96658811657337,
-4.78316238877312));
#365336=CARTESIAN_POINT('Ctrl Pts',(-0.0484699606159579,-2.02317940049164,
-4.8436197561483));
#365337=CARTESIAN_POINT('Ctrl Pts',(-0.570341982644288,-1.94138567221422,
-4.90407497831006));
#365338=CARTESIAN_POINT('Ctrl Pts',(-1.05344257214943,-1.72773301391037,
-4.96439238877312));
#365339=CARTESIAN_POINT('Ctrl Pts',(-1.46487731147995,-1.39633043580918,
-5.02484975614831));
#365340=CARTESIAN_POINT('Ctrl Pts',(-1.77605965724426,-0.969474290197928,
-5.08530497831004));
#365341=CARTESIAN_POINT('Ctrl Pts',(-1.96658811657335,-0.476795343858433,
-5.14562238877313));
#365342=CARTESIAN_POINT('Ctrl Pts',(-2.02317940049163,0.0484699606159606,
-5.2060797561483));
#365343=CARTESIAN_POINT('Ctrl Pts',(-1.94138567221425,0.570341982644311,
-5.26653497831003));
#365344=CARTESIAN_POINT('Ctrl Pts',(-1.72773301391036,1.05344257214944,
-5.32685238877313));
#365345=CARTESIAN_POINT('Ctrl Pts',(-1.39633043580918,1.46487731147996,
-5.3873097561483));
#365346=CARTESIAN_POINT('Ctrl Pts',(-0.969474290197916,1.77605965724424,
-5.44776497831006));
#365347=CARTESIAN_POINT('Ctrl Pts',(-0.476795343858422,1.96658811657339,
-5.5080823887731));
#365348=CARTESIAN_POINT('Ctrl Pts',(0.0484699606159706,2.02317940049163,
-5.56853975614829));
#365349=CARTESIAN_POINT('Ctrl Pts',(0.570341982644291,1.94138567221422,
-5.62899497831007));
#365350=CARTESIAN_POINT('Ctrl Pts',(1.05344257214944,1.72773301391032,-5.68931238877313));
#365351=CARTESIAN_POINT('Ctrl Pts',(1.46487731147996,1.3963304358092,-5.74976975614823));
#365352=CARTESIAN_POINT('Ctrl Pts',(1.77605965724441,0.969474290197947,
-5.81022497831013));
#365353=CARTESIAN_POINT('Ctrl Pts',(1.96658811657315,0.476795343858267,
-5.87054238877304));
#365354=CARTESIAN_POINT('Ctrl Pts',(2.02317940049197,-0.0484699606151168,
-5.93099975614826));
#365355=CARTESIAN_POINT('Ctrl Pts',(1.94138567221262,-0.570341982647331,
-5.99145497831012));
#365356=CARTESIAN_POINT('Ctrl Pts',(1.72773301391079,-1.05344257214282,
-6.05177238877488));
#365357=CARTESIAN_POINT('Ctrl Pts',(1.39633043583791,-1.46487731150212,
-6.1122297561358));
#365358=CARTESIAN_POINT('Ctrl Pts',(0.969474290103704,-1.77605965719443,
-6.17268497832268));
#365359=CARTESIAN_POINT('Ctrl Pts',(0.476795344014053,-1.96658811647506,
-6.23300238886911));
#365360=CARTESIAN_POINT('Ctrl Pts',(-0.0484699607888847,-2.02317940162764,
-6.293459755551));
#365361=CARTESIAN_POINT('Ctrl Pts',(-0.570341982515374,-1.94138566986718,
-6.35391497894857));
#365362=CARTESIAN_POINT('Ctrl Pts',(-1.0534425689941,-1.72773301427299,
-6.41423239105532));
#365363=CARTESIAN_POINT('Ctrl Pts',(-1.46487733129139,-1.39633044764682,
-6.47468974174144));
#365364=CARTESIAN_POINT('Ctrl Pts',(-1.77605962440754,-0.969474272408487,
-6.53514499410053));
#365365=CARTESIAN_POINT('Ctrl Pts',(-1.96658808441403,-0.4767953693466,
-6.59546242507117));
#365366=CARTESIAN_POINT('Ctrl Pts',(-2.02317971788315,0.0484700612956726,
-6.65591951867769));
#365367=CARTESIAN_POINT('Ctrl Pts',(-1.94138529374751,0.57034175258804,
-6.71637524065362));
#365368=CARTESIAN_POINT('Ctrl Pts',(-1.7277327906675,1.05344225923825,-6.77669281345839));
#365369=CARTESIAN_POINT('Ctrl Pts',(-1.39633190064527,1.46488023063332,
-6.83714685373563));
#365370=CARTESIAN_POINT('Ctrl Pts',(-0.969474795144666,1.77605674551469,
-6.89760831895014));
#365371=CARTESIAN_POINT('Ctrl Pts',(-0.476792483974202,1.96658170561334,
-6.95792512927773));
#365372=CARTESIAN_POINT('Ctrl Pts',(0.0484734593030573,2.0232081210323,
-7.01835708981697));
#365373=CARTESIAN_POINT('Ctrl Pts',(0.570336624689882,1.94136175768686,
-7.07885725203471));
#365374=CARTESIAN_POINT('Ctrl Pts',(1.05340619968671,1.72778052727257,-7.13918044053492));
#365375=CARTESIAN_POINT('Ctrl Pts',(1.46503146071072,1.39600002911185,-7.19942807213429));
#365376=CARTESIAN_POINT('Ctrl Pts',(1.77572739170825,0.970967789756964,
-7.26046972816476));
#365377=CARTESIAN_POINT('Ctrl Pts',(1.9679960876878,0.471734127632586,-7.31921124624962));
#365378=CARTESIAN_POINT('Ctrl Pts',(2.00016367750205,0.139563645186354,
-7.36277016686196));
#365379=CARTESIAN_POINT('Ctrl Pts',(2.00016367750204,-0.0349606549172864,
-7.37954989315336));
#365380=CARTESIAN_POINT('Ctrl Pts',(1.20005141796495,-0.0349598558146385,
-1.58019721042982));
#365381=CARTESIAN_POINT('Ctrl Pts',(1.20005141796495,-0.196639509400045,
-1.59574198174499));
#365382=CARTESIAN_POINT('Ctrl Pts',(1.15732797686238,-0.340816716447164,
-1.6447382432052));
#365383=CARTESIAN_POINT('Ctrl Pts',(1.02794595474197,-0.654182454634222,
-1.70085757593186));
#365384=CARTESIAN_POINT('Ctrl Pts',(0.824371570064879,-0.890750973398493,
-1.76298366242172));
#365385=CARTESIAN_POINT('Ctrl Pts',(0.563969291479731,-1.07614468532721,
-1.82314153495176));
#365386=CARTESIAN_POINT('Ctrl Pts',(0.268053015090469,-1.18466145511491,
-1.88305373693166));
#365387=CARTESIAN_POINT('Ctrl Pts',(-0.0484395870237313,-1.21410753423567,
-1.9438363016732));
#365388=CARTESIAN_POINT('Ctrl Pts',(-0.361651032204537,-1.15949959431507,
-2.00439370017114));
#365389=CARTESIAN_POINT('Ctrl Pts',(-0.648204859882796,-1.02726348852071,
-2.06435695179187));
#365390=CARTESIAN_POINT('Ctrl Pts',(-0.892791267502041,-0.824210832808723,
-2.12500826054469));
#365391=CARTESIAN_POINT('Ctrl Pts',(-1.07560894612736,-0.564190577762509,
-2.18562659547641));
#365392=CARTESIAN_POINT('Ctrl Pts',(-1.1847293912525,-0.268030428045687,
-2.24559800960236));
#365393=CARTESIAN_POINT('Ctrl Pts',(-1.21410751416084,0.0484963826130714,
-2.30623010797513));
#365394=CARTESIAN_POINT('Ctrl Pts',(-1.1595132046369,0.36162639690026,-2.36685750692005));
#365395=CARTESIAN_POINT('Ctrl Pts',(-1.02725604518277,0.648203827608334,
-2.42682890216184));
#365396=CARTESIAN_POINT('Ctrl Pts',(-0.824211659423609,0.892796064601774,
-2.48745940373019));
#365397=CARTESIAN_POINT('Ctrl Pts',(-0.564191142051916,1.07560808882016,
-2.54808760329284));
#365398=CARTESIAN_POINT('Ctrl Pts',(-0.268030403610479,1.18472901687534,
-2.60805895542665));
#365399=CARTESIAN_POINT('Ctrl Pts',(0.0484964956129267,1.21410782343574,
-2.66868935921047));
#365400=CARTESIAN_POINT('Ctrl Pts',(0.361626396132377,1.15951315047799,
-2.72931761037603));
#365401=CARTESIAN_POINT('Ctrl Pts',(0.648203803824844,1.0272560382112,-2.78928895746987));
#365402=CARTESIAN_POINT('Ctrl Pts',(0.892796076188025,0.824211675103123,
-2.84991935728737));
#365403=CARTESIAN_POINT('Ctrl Pts',(1.07560808862158,0.56419113400383,-2.91054761072926));
#365404=CARTESIAN_POINT('Ctrl Pts',(1.18472901588199,0.26803040550146,-2.97051895749492));
#365405=CARTESIAN_POINT('Ctrl Pts',(1.21410782431058,-0.0484964950668307,
-3.03114935724649));
#365406=CARTESIAN_POINT('Ctrl Pts',(1.15951315008857,-0.361626396645578,
-3.09177761073831));
#365407=CARTESIAN_POINT('Ctrl Pts',(1.02725603829716,-0.6482038036989,-3.15174895749339));
#365408=CARTESIAN_POINT('Ctrl Pts',(0.824211675135244,-0.892796076188428,
-3.21237935724692));
#365409=CARTESIAN_POINT('Ctrl Pts',(0.564191133978922,-1.07560808862653,
-3.27300761073802));
#365410=CARTESIAN_POINT('Ctrl Pts',(0.268030405508416,-1.18472901588096,
-3.33297895749366));
#365411=CARTESIAN_POINT('Ctrl Pts',(-0.0484964950686988,-1.21410782431092,
-3.39360935724675));
#365412=CARTESIAN_POINT('Ctrl Pts',(-0.361626396644909,-1.15951315008879,
-3.45423761073805));
#365413=CARTESIAN_POINT('Ctrl Pts',(-0.648203803698724,-1.02725603829705,
-3.51420895749367));
#365414=CARTESIAN_POINT('Ctrl Pts',(-0.89279607618879,-0.824211675135025,
-3.57483935724674));
#365415=CARTESIAN_POINT('Ctrl Pts',(-1.07560808862643,-0.564191133979103,
-3.63546761073801));
#365416=CARTESIAN_POINT('Ctrl Pts',(-1.18472901588094,-0.26803040550839,
-3.6954389574937));
#365417=CARTESIAN_POINT('Ctrl Pts',(-1.21410782431094,0.0484964950687397,
-3.75606935724672));
#365418=CARTESIAN_POINT('Ctrl Pts',(-1.1595131500888,0.361626396644898,
-3.81669761073803));
#365419=CARTESIAN_POINT('Ctrl Pts',(-1.02725603829704,0.648203803698727,
-3.87666895749368));
#365420=CARTESIAN_POINT('Ctrl Pts',(-0.824211675135021,0.892796076188792,
-3.93729935724673));
#365421=CARTESIAN_POINT('Ctrl Pts',(-0.564191133979095,1.07560808862643,
-3.99792761073801));
#365422=CARTESIAN_POINT('Ctrl Pts',(-0.268030405508389,1.18472901588092,
-4.05789895749373));
#365423=CARTESIAN_POINT('Ctrl Pts',(0.0484964950687464,1.21410782431094,
-4.11852935724671));
#365424=CARTESIAN_POINT('Ctrl Pts',(0.3616263966449,1.15951315008879,-4.17915761073805));
#365425=CARTESIAN_POINT('Ctrl Pts',(0.648203803698728,1.02725603829704,
-4.23912895749368));
#365426=CARTESIAN_POINT('Ctrl Pts',(0.892796076188791,0.824211675135014,
-4.29975935724674));
#365427=CARTESIAN_POINT('Ctrl Pts',(1.07560808862644,0.564191133979099,
-4.36038761073799));
#365428=CARTESIAN_POINT('Ctrl Pts',(1.18472901588094,0.268030405508375,
-4.42035895749369));
#365429=CARTESIAN_POINT('Ctrl Pts',(1.21410782431093,-0.0484964950687469,
-4.48098935724673));
#365430=CARTESIAN_POINT('Ctrl Pts',(1.15951315008879,-0.361626396644902,
-4.54161761073803));
#365431=CARTESIAN_POINT('Ctrl Pts',(1.02725603829703,-0.648203803698725,
-4.6015889574937));
#365432=CARTESIAN_POINT('Ctrl Pts',(0.824211675135013,-0.892796076188798,
-4.66221935724673));
#365433=CARTESIAN_POINT('Ctrl Pts',(0.564191133979094,-1.07560808862644,
-4.722847610738));
#365434=CARTESIAN_POINT('Ctrl Pts',(0.268030405508374,-1.18472901588094,
-4.7828189574937));
#365435=CARTESIAN_POINT('Ctrl Pts',(-0.04849649506876,-1.21410782431095,
-4.84344935724668));
#365436=CARTESIAN_POINT('Ctrl Pts',(-0.361626396644897,-1.15951315008877,
-4.90407761073806));
#365437=CARTESIAN_POINT('Ctrl Pts',(-0.648203803698715,-1.02725603829702,
-4.96404895749372));
#365438=CARTESIAN_POINT('Ctrl Pts',(-0.892796076188803,-0.824211675135015,
-5.02467935724671));
#365439=CARTESIAN_POINT('Ctrl Pts',(-1.07560808862644,-0.564191133979088,
-5.085307610738));
#365440=CARTESIAN_POINT('Ctrl Pts',(-1.18472901588092,-0.268030405508372,
-5.14527895749374));
#365441=CARTESIAN_POINT('Ctrl Pts',(-1.21410782431095,0.0484964950687572,
-5.20590935724669));
#365442=CARTESIAN_POINT('Ctrl Pts',(-1.1595131500888,0.361626396644921,
-5.26653761073799));
#365443=CARTESIAN_POINT('Ctrl Pts',(-1.02725603829702,0.64820380369872,
-5.32650895749373));
#365444=CARTESIAN_POINT('Ctrl Pts',(-0.824211675135014,0.892796076188816,
-5.38713935724669));
#365445=CARTESIAN_POINT('Ctrl Pts',(-0.564191133979076,1.07560808862641,
-5.44776761073806));
#365446=CARTESIAN_POINT('Ctrl Pts',(-0.268030405508379,1.18472901588095,
-5.50773895749365));
#365447=CARTESIAN_POINT('Ctrl Pts',(0.0484964950687955,1.21410782431095,
-5.56836935724668));
#365448=CARTESIAN_POINT('Ctrl Pts',(0.361626396644923,1.15951315008874,
-5.62899761073811));
#365449=CARTESIAN_POINT('Ctrl Pts',(0.648203803698529,1.02725603829711,
-5.68896895749371));
#365450=CARTESIAN_POINT('Ctrl Pts',(0.892796076189156,0.824211675134774,
-5.74959935724652));
#365451=CARTESIAN_POINT('Ctrl Pts',(1.07560808862635,0.564191133979143,
-5.81022761073827));
#365452=CARTESIAN_POINT('Ctrl Pts',(1.18472901588091,0.268030405509044,
-5.87019895749336));
#365453=CARTESIAN_POINT('Ctrl Pts',(1.2141078243105,-0.0484964950705043,
-5.93082935724695));
#365454=CARTESIAN_POINT('Ctrl Pts',(1.15951315009036,-0.361626396638523,
-5.99145761073686));
#365455=CARTESIAN_POINT('Ctrl Pts',(1.02725603828656,-0.648203803720622,
-6.05142895750248));
#365456=CARTESIAN_POINT('Ctrl Pts',(0.824211675164934,-0.892796076174764,
-6.11205935720599));
#365457=CARTESIAN_POINT('Ctrl Pts',(0.564191134059871,-1.07560808852829,
-6.17268761076101));
#365458=CARTESIAN_POINT('Ctrl Pts',(0.268030404959908,-1.18472901600022,
-6.23265895786053));
#365459=CARTESIAN_POINT('Ctrl Pts',(-0.048496494303855,-1.21410782509991,
-6.29328935527559));
#365460=CARTESIAN_POINT('Ctrl Pts',(-0.361626395111129,-1.15951314891753,
-6.35391761278417));
#365461=CARTESIAN_POINT('Ctrl Pts',(-0.648203807785757,-1.02725603400328,
-6.41388896506857));
#365462=CARTESIAN_POINT('Ctrl Pts',(-0.892796086148053,-0.82421169457497,
-6.47451931057689));
#365463=CARTESIAN_POINT('Ctrl Pts',(-1.0756080601232,-0.564191117561312,
-6.53514766561185));
#365464=CARTESIAN_POINT('Ctrl Pts',(-1.18472898053544,-0.268030410347432,
-6.59511906407632));
#365465=CARTESIAN_POINT('Ctrl Pts',(-1.21410817056974,0.0484965775982433,
-6.65574860156863));
#365466=CARTESIAN_POINT('Ctrl Pts',(-1.15951264802113,0.361626359829526,
-6.71637855817043));
#365467=CARTESIAN_POINT('Ctrl Pts',(-1.02725631549215,0.648202679709777,
-6.77634998994504));
#365468=CARTESIAN_POINT('Ctrl Pts',(-0.824212514048729,0.89279989750689,
-6.83697046026166));
#365469=CARTESIAN_POINT('Ctrl Pts',(-0.564185827571163,1.07561000588125,
-6.89761936594616));
#365470=CARTESIAN_POINT('Ctrl Pts',(-0.268055236457238,1.1847006164406,
-6.95758396792716));
#365471=CARTESIAN_POINT('Ctrl Pts',(0.0485472352404887,1.2142038916925,
-7.01813896161907));
#365472=CARTESIAN_POINT('Ctrl Pts',(0.361655804485534,1.15924149264237,
-7.07893382111904));
#365473=CARTESIAN_POINT('Ctrl Pts',(0.6478968782727,1.02825270748,-7.1387952204064));
#365474=CARTESIAN_POINT('Ctrl Pts',(0.893414088159582,0.820656810820771,
-7.19914743650299));
#365475=CARTESIAN_POINT('Ctrl Pts',(1.07501647976632,0.576321349623175,
-7.26054245691513));
#365476=CARTESIAN_POINT('Ctrl Pts',(1.18621324528802,0.224452404214759,
-7.3192609169548));
#365477=CARTESIAN_POINT('Ctrl Pts',(1.20016374408797,0.152327073866745,
-7.36128002094695));
#365478=CARTESIAN_POINT('Ctrl Pts',(1.20016374408796,-0.0349890780536599,
-7.37928962624155));
#365479=CARTESIAN_POINT('Ctrl Pts',(1.19994860179671,0.0349330361207006,
-2.22019720516939));
#365480=CARTESIAN_POINT('Ctrl Pts',(1.19994860179671,-0.126746617464705,
-2.23574197648456));
#365481=CARTESIAN_POINT('Ctrl Pts',(1.18628451104366,-0.235287042882826,
-2.2810964912132));
#365482=CARTESIAN_POINT('Ctrl Pts',(1.07477771342961,-0.573169099315595,
-2.33867755519319));
#365483=CARTESIAN_POINT('Ctrl Pts',(0.893209191596192,-0.821391071780957,
-2.40041325450729));
#365484=CARTESIAN_POINT('Ctrl Pts',(0.647719578695754,-1.02788019949386,
-2.46067439994995));
#365485=CARTESIAN_POINT('Ctrl Pts',(0.361523604188232,-1.15911171219588,
-2.52056034931245));
#365486=CARTESIAN_POINT('Ctrl Pts',(0.0484713603287608,-1.21397018964645,
-2.58134810525369));
#365487=CARTESIAN_POINT('Ctrl Pts',(-0.26807499252822,-1.18447453220047,
-2.64190541780525));
#365488=CARTESIAN_POINT('Ctrl Pts',(-0.564145022724671,-1.07538119354467,
-2.70186948165707));
#365489=CARTESIAN_POINT('Ctrl Pts',(-0.82411227040745,-0.892592747940269,
-2.76251800818134));
#365490=CARTESIAN_POINT('Ctrl Pts',(-1.02710741719481,-0.648025648702113,
-2.82313903087394));
#365491=CARTESIAN_POINT('Ctrl Pts',(-1.15932278442025,-0.361494315792975,
-2.88311038111178));
#365492=CARTESIAN_POINT('Ctrl Pts',(-1.21389060301799,-0.0484207535259056,
-2.94373983918878));
#365493=CARTESIAN_POINT('Ctrl Pts',(-1.18449856839689,0.268050248144059,
-3.00436996521972));
#365494=CARTESIAN_POINT('Ctrl Pts',(-1.0753804241319,0.564150242879215,
-3.06434127064474));
#365495=CARTESIAN_POINT('Ctrl Pts',(-0.892588631186338,0.824111463629319,
-3.12496913072614));
#365496=CARTESIAN_POINT('Ctrl Pts',(-0.648026852820059,1.02710713661446,
-3.18560006416148));
#365497=CARTESIAN_POINT('Ctrl Pts',(-0.361494335707408,1.15932328272349,
-3.24557132342766));
#365498=CARTESIAN_POINT('Ctrl Pts',(-0.0484206753242147,1.21389025844596,
-3.30619908602272));
#365499=CARTESIAN_POINT('Ctrl Pts',(0.268050244650624,1.18449860355023,
-3.36683007137514));
#365500=CARTESIAN_POINT('Ctrl Pts',(0.564150258467979,1.07538045277468,
-3.42680132544561));
#365501=CARTESIAN_POINT('Ctrl Pts',(0.824111444426381,0.892588621200653,
-3.48742908409296));
#365502=CARTESIAN_POINT('Ctrl Pts',(1.02710714086036,0.648026848734914,
-3.54806007173318));
#365503=CARTESIAN_POINT('Ctrl Pts',(1.15932328389686,0.361494337262554,
-3.60803132546964));
#365504=CARTESIAN_POINT('Ctrl Pts',(1.21389025765669,0.0484206760863054,
-3.66865908405205));
#365505=CARTESIAN_POINT('Ctrl Pts',(1.18449860343075,-0.268050245199621,
-3.72929007174227));
#365506=CARTESIAN_POINT('Ctrl Pts',(1.07538045287309,-0.564150258386447,
-3.78926132546809));
#365507=CARTESIAN_POINT('Ctrl Pts',(0.892588621215019,-0.824111444396376,
-3.84988908405249));
#365508=CARTESIAN_POINT('Ctrl Pts',(0.648026848712835,-1.02710714087089,
-3.91052007174198));
#365509=CARTESIAN_POINT('Ctrl Pts',(0.361494337268959,-1.15932328389524,
-3.97049132546837));
#365510=CARTESIAN_POINT('Ctrl Pts',(0.0484206760845926,-1.21389025765713,
-4.03111908405232));
#365511=CARTESIAN_POINT('Ctrl Pts',(-0.268050245198952,-1.18449860343081,
-4.09175007174202));
#365512=CARTESIAN_POINT('Ctrl Pts',(-0.564150258386389,-1.07538045287319,
-4.15172132546838));
#365513=CARTESIAN_POINT('Ctrl Pts',(-0.82411144439661,-0.892588621214665,
-4.2123490840523));
#365514=CARTESIAN_POINT('Ctrl Pts',(-1.0271071408708,-0.648026848713027,
-4.27298007174198));
#365515=CARTESIAN_POINT('Ctrl Pts',(-1.15932328389526,-0.361494337268938,
-4.33295132546841));
#365516=CARTESIAN_POINT('Ctrl Pts',(-1.21389025765712,-0.0484206760845532,
-4.39357908405229));
#365517=CARTESIAN_POINT('Ctrl Pts',(-1.1844986034308,0.268050245198939,
-4.45421007174199));
#365518=CARTESIAN_POINT('Ctrl Pts',(-1.07538045287319,0.564150258386394,
-4.51418132546839));
#365519=CARTESIAN_POINT('Ctrl Pts',(-0.892588621214658,0.82411144439661,
-4.5748090840523));
#365520=CARTESIAN_POINT('Ctrl Pts',(-0.648026848713022,1.0271071408708,
-4.63544007174198));
#365521=CARTESIAN_POINT('Ctrl Pts',(-0.361494337268941,1.15932328389527,
-4.69541132546844));
#365522=CARTESIAN_POINT('Ctrl Pts',(-0.0484206760845442,1.21389025765711,
-4.75603908405227));
#365523=CARTESIAN_POINT('Ctrl Pts',(0.268050245198942,1.18449860343081,
-4.81667007174201));
#365524=CARTESIAN_POINT('Ctrl Pts',(0.564150258386395,1.07538045287318,
-4.87664132546839));
#365525=CARTESIAN_POINT('Ctrl Pts',(0.824111444396615,0.892588621214655,
-4.9372690840523));
#365526=CARTESIAN_POINT('Ctrl Pts',(1.02710714087079,0.648026848713006,
-4.99790007174195));
#365527=CARTESIAN_POINT('Ctrl Pts',(1.15932328389525,0.361494337268927,
-5.0578713254684));
#365528=CARTESIAN_POINT('Ctrl Pts',(1.21389025765711,0.0484206760845428,
-5.11849908405229));
#365529=CARTESIAN_POINT('Ctrl Pts',(1.1844986034308,-0.268050245198941,
-5.179130071742));
#365530=CARTESIAN_POINT('Ctrl Pts',(1.07538045287319,-0.5641502583864,-5.2391013254684));
#365531=CARTESIAN_POINT('Ctrl Pts',(0.892588621214648,-0.824111444396615,
-5.29972908405229));
#365532=CARTESIAN_POINT('Ctrl Pts',(0.648026848713012,-1.0271071408708,
-5.36036007174197));
#365533=CARTESIAN_POINT('Ctrl Pts',(0.361494337268925,-1.15932328389526,
-5.42033132546841));
#365534=CARTESIAN_POINT('Ctrl Pts',(0.0484206760845338,-1.21389025765709,
-5.48095908405224));
#365535=CARTESIAN_POINT('Ctrl Pts',(-0.268050245198938,-1.18449860343081,
-5.54159007174203));
#365536=CARTESIAN_POINT('Ctrl Pts',(-0.564150258386406,-1.0753804528732,
-5.60156132546843));
#365537=CARTESIAN_POINT('Ctrl Pts',(-0.824111444396613,-0.89258862121464,
-5.66218908405228));
#365538=CARTESIAN_POINT('Ctrl Pts',(-1.02710714087079,-0.648026848713008,
-5.72282007174197));
#365539=CARTESIAN_POINT('Ctrl Pts',(-1.15932328389528,-0.36149433726893,
-5.78279132546845));
#365540=CARTESIAN_POINT('Ctrl Pts',(-1.2138902576571,-0.0484206760845329,
-5.84341908405225));
#365541=CARTESIAN_POINT('Ctrl Pts',(-1.18449860343078,0.268050245198954,
-5.90405007174196));
#365542=CARTESIAN_POINT('Ctrl Pts',(-1.07538045287319,0.564150258386408,
-5.96402132546844));
#365543=CARTESIAN_POINT('Ctrl Pts',(-0.892588621214629,0.824111444396606,
-6.02464908405225));
#365544=CARTESIAN_POINT('Ctrl Pts',(-0.64802684871302,1.02710714087081,
-6.08528007174203));
#365545=CARTESIAN_POINT('Ctrl Pts',(-0.361494337268917,1.15932328389523,
-6.14525132546836));
#365546=CARTESIAN_POINT('Ctrl Pts',(-0.048420676084498,1.21389025765709,
-6.20587908405224));
#365547=CARTESIAN_POINT('Ctrl Pts',(0.268050245198975,1.18449860343083,
-6.26651007174208));
#365548=CARTESIAN_POINT('Ctrl Pts',(0.564150258386226,1.07538045287327,
-6.32648132546841));
#365549=CARTESIAN_POINT('Ctrl Pts',(0.824111444396827,0.892588621214275,
-6.38710908405208));
#365550=CARTESIAN_POINT('Ctrl Pts',(1.0271071408709,0.648026848713156,-6.44774007174223));
#365551=CARTESIAN_POINT('Ctrl Pts',(1.159323283895,0.361494337269589,-6.50771132546807));
#365552=CARTESIAN_POINT('Ctrl Pts',(1.21389025765673,0.0484206760826282,
-6.56833908405251));
#365553=CARTESIAN_POINT('Ctrl Pts',(1.18449860343187,-0.268050245192022,
-6.62897007174084));
#365554=CARTESIAN_POINT('Ctrl Pts',(1.07538045286828,-0.564150258411146,
-6.68894132547714));
#365555=CARTESIAN_POINT('Ctrl Pts',(0.892588621213993,-0.824111444364615,
-6.74956908401155));
#365556=CARTESIAN_POINT('Ctrl Pts',(0.648026848838496,-1.0271071407854,
-6.81020007176602));
#365557=CARTESIAN_POINT('Ctrl Pts',(0.361494336755823,-1.1593232842844,
-6.87017132583052));
#365558=CARTESIAN_POINT('Ctrl Pts',(0.0484206766338695,-1.2138902567815,
-6.93079908208711));
#365559=CARTESIAN_POINT('Ctrl Pts',(-0.268050243328471,-1.18449860442843,
-6.99143007381518));
#365560=CARTESIAN_POINT('Ctrl Pts',(-0.564150266443273,-1.07538045302616,
-7.05140133291083));
#365561=CARTESIAN_POINT('Ctrl Pts',(-0.824111428662813,-0.892588609834598,
-7.11202903755537));
#365562=CARTESIAN_POINT('Ctrl Pts',(-1.02710714802879,-0.648026871740004,
-7.17266012714546));
#365563=CARTESIAN_POINT('Ctrl Pts',(-1.15932333812035,-0.361494339370128,
-7.23263142938285));
#365564=CARTESIAN_POINT('Ctrl Pts',(-1.21388994830272,-0.048420558641127,
-7.29325833250989));
#365565=CARTESIAN_POINT('Ctrl Pts',(-1.18449897688191,0.268050252868152,
-7.3538910230542));
#365566=CARTESIAN_POINT('Ctrl Pts',(-1.07538131032931,0.564149776786355,
-7.41386233272661));
#365567=CARTESIAN_POINT('Ctrl Pts',(-0.89258382755218,0.824110299740277,
-7.47448020435212));
#365568=CARTESIAN_POINT('Ctrl Pts',(-0.648027824318076,1.02711576339274,
-7.53513199456933));
#365569=CARTESIAN_POINT('Ctrl Pts',(-0.361519103800307,1.1593054263198,
-7.59509558925458));
#365570=CARTESIAN_POINT('Ctrl Pts',(-0.048363558710048,1.21390597518738,
-7.65565075634608));
#365571=CARTESIAN_POINT('Ctrl Pts',(0.268072537684821,1.18437146807072,
-7.71644050362745));
#365572=CARTESIAN_POINT('Ctrl Pts',(0.563930411939142,1.07613883654808,
-7.77632820376135));
#365573=CARTESIAN_POINT('Ctrl Pts',(0.82426225220675,0.889715887308659,
-7.83657609568004));
#365574=CARTESIAN_POINT('Ctrl Pts',(1.02783344969258,0.657090690457504,
-7.89836582380498));
#365575=CARTESIAN_POINT('Ctrl Pts',(1.15670010462145,0.329911052415485,
-7.95561053869555));
#365576=CARTESIAN_POINT('Ctrl Pts',(1.19983645566974,0.222219960564689,
-8.00127996772839));
#365577=CARTESIAN_POINT('Ctrl Pts',(1.19983645566973,0.0349038086442839,
-8.01928957302298));
#365578=CARTESIAN_POINT('Ctrl Pts',(1.99994859520949,0.0349419760186855,
-2.22027906663631));
#365579=CARTESIAN_POINT('Ctrl Pts',(1.99994859520949,-0.133161143166691,
-2.23644142527053));
#365580=CARTESIAN_POINT('Ctrl Pts',(1.96833139354662,-0.472425718114294,
-2.28062587414611));
#365581=CARTESIAN_POINT('Ctrl Pts',(1.77549751488388,-0.970378153502274,
-2.33932132964638));
#365582=CARTESIAN_POINT('Ctrl Pts',(1.46486827473653,-1.39599810161593,
-2.40041168228136));
#365583=CARTESIAN_POINT('Ctrl Pts',(1.0532724675317,-1.72756949816,-2.46064650153962));
#365584=CARTESIAN_POINT('Ctrl Pts',(0.570253827701872,-1.94116844962337,
-2.52097328730337));
#365585=CARTESIAN_POINT('Ctrl Pts',(0.0484505622703552,-2.02298787581022,
-2.58147196284819));
#365586=CARTESIAN_POINT('Ctrl Pts',(-0.476762817249676,-1.96636546213765,
-2.64190473727344));
#365587=CARTESIAN_POINT('Ctrl Pts',(-0.969389646094711,-1.7758542783469,
-2.70222141276452));
#365588=CARTESIAN_POINT('Ctrl Pts',(-1.39619412835269,-1.46471035101601,
-2.76268238970025));
#365589=CARTESIAN_POINT('Ctrl Pts',(-1.72755848446788,-1.05330968911041,
-2.8231370123091));
#365590=CARTESIAN_POINT('Ctrl Pts',(-1.94118200928605,-0.570259037663673,
-2.88345449584336));
#365591=CARTESIAN_POINT('Ctrl Pts',(-2.02296215046454,-0.0484473116516587,
-2.94390972032538));
#365592=CARTESIAN_POINT('Ctrl Pts',(-1.96637109382515,0.476765855935366,
-3.00436740295728));
#365593=CARTESIAN_POINT('Ctrl Pts',(-1.77585739520295,0.969389009874219,
-3.06468474103924));
#365594=CARTESIAN_POINT('Ctrl Pts',(-1.46470740175196,1.39619269138418,
-3.12513949735647));
#365595=CARTESIAN_POINT('Ctrl Pts',(-1.05331000180424,1.72755870986409,
-3.18559743702838));
#365596=CARTESIAN_POINT('Ctrl Pts',(-0.570259275444307,1.94118238224882,
-3.2459147561141));
#365597=CARTESIAN_POINT('Ctrl Pts',(-0.0484472107178668,2.02296183497224,
-3.30636948355066));
#365598=CARTESIAN_POINT('Ctrl Pts',(0.476765831354286,1.96637112545875,
-3.36682743921798));
#365599=CARTESIAN_POINT('Ctrl Pts',(0.969389026744113,1.77585742843582,
-3.42714475673536));
#365600=CARTESIAN_POINT('Ctrl Pts',(1.39619267971627,1.46470738191116,-3.48759948296635));
#365601=CARTESIAN_POINT('Ctrl Pts',(1.72755870948907,1.05331000492523,-3.54805743931225));
#365602=CARTESIAN_POINT('Ctrl Pts',(1.9411823845861,0.570259275622033,-3.60837475674778));
#365603=CARTESIAN_POINT('Ctrl Pts',(2.02296183383815,0.0484472105365179,
-3.66882948295392));
#365604=CARTESIAN_POINT('Ctrl Pts',(1.96637112555601,-0.476765831198158,
-3.72928743931407));
#365605=CARTESIAN_POINT('Ctrl Pts',(1.77585742848668,-0.969389026837108,
-3.78960475674772));
#365606=CARTESIAN_POINT('Ctrl Pts',(1.46470738188885,-1.39619267968778,
-3.85005948295395));
#365607=CARTESIAN_POINT('Ctrl Pts',(1.05331000493188,-1.72755870948857,
-3.910517439314));
#365608=CARTESIAN_POINT('Ctrl Pts',(0.570259275619007,-1.9411823845877,
-3.97083475674782));
#365609=CARTESIAN_POINT('Ctrl Pts',(0.0484472105373659,-2.02296183383781,
-4.03128948295388));
#365610=CARTESIAN_POINT('Ctrl Pts',(-0.476765831198311,-1.96637112555626,
-4.09174743931402));
#365611=CARTESIAN_POINT('Ctrl Pts',(-0.969389026837092,-1.77585742848654,
-4.15206475674782));
#365612=CARTESIAN_POINT('Ctrl Pts',(-1.39619267968775,-1.46470738188883,
-4.21251948295388));
#365613=CARTESIAN_POINT('Ctrl Pts',(-1.72755870948862,-1.05331000493188,
-4.27297743931401));
#365614=CARTESIAN_POINT('Ctrl Pts',(-1.94118238458768,-0.570259275619005,
-4.33329475674783));
#365615=CARTESIAN_POINT('Ctrl Pts',(-2.0229618338378,-0.0484472105373586,
-4.39374948295387));
#365616=CARTESIAN_POINT('Ctrl Pts',(-1.96637112555625,0.476765831198322,
-4.45420743931402));
#365617=CARTESIAN_POINT('Ctrl Pts',(-1.77585742848654,0.969389026837096,
-4.51452475674782));
#365618=CARTESIAN_POINT('Ctrl Pts',(-1.46470738188882,1.39619267968775,
-4.57497948295388));
#365619=CARTESIAN_POINT('Ctrl Pts',(-1.05331000493187,1.72755870948862,
-4.63543743931401));
#365620=CARTESIAN_POINT('Ctrl Pts',(-0.570259275619004,1.9411823845877,
-4.69575475674784));
#365621=CARTESIAN_POINT('Ctrl Pts',(-0.0484472105373471,2.0229618338378,
-4.75620948295387));
#365622=CARTESIAN_POINT('Ctrl Pts',(0.476765831198326,1.96637112555626,
-4.81666743931402));
#365623=CARTESIAN_POINT('Ctrl Pts',(0.969389026837101,1.77585742848653,
-4.87698475674782));
#365624=CARTESIAN_POINT('Ctrl Pts',(1.39619267968776,1.46470738188882,-4.93743948295388));
#365625=CARTESIAN_POINT('Ctrl Pts',(1.72755870948861,1.05331000493185,-4.997897439314));
#365626=CARTESIAN_POINT('Ctrl Pts',(1.94118238458768,0.570259275618993,
-5.05821475674782));
#365627=CARTESIAN_POINT('Ctrl Pts',(2.0229618338378,0.0484472105373451,
-5.11866948295387));
#365628=CARTESIAN_POINT('Ctrl Pts',(1.96637112555625,-0.476765831198331,
-5.17912743931402));
#365629=CARTESIAN_POINT('Ctrl Pts',(1.77585742848654,-0.969389026837107,
-5.23944475674783));
#365630=CARTESIAN_POINT('Ctrl Pts',(1.46470738188881,-1.39619267968776,
-5.29989948295387));
#365631=CARTESIAN_POINT('Ctrl Pts',(1.05331000493185,-1.72755870948862,
-5.36035743931401));
#365632=CARTESIAN_POINT('Ctrl Pts',(0.57025927561899,-1.94118238458768,
-5.42067475674783));
#365633=CARTESIAN_POINT('Ctrl Pts',(0.0484472105373359,-2.02296183383778,
-5.48112948295386));
#365634=CARTESIAN_POINT('Ctrl Pts',(-0.476765831198329,-1.96637112555626,
-5.54158743931402));
#365635=CARTESIAN_POINT('Ctrl Pts',(-0.96938902683712,-1.77585742848655,
-5.60190475674783));
#365636=CARTESIAN_POINT('Ctrl Pts',(-1.39619267968776,-1.4647073818888,
-5.66235948295387));
#365637=CARTESIAN_POINT('Ctrl Pts',(-1.72755870948862,-1.05331000493185,
-5.722817439314));
#365638=CARTESIAN_POINT('Ctrl Pts',(-1.9411823845877,-0.570259275618991,
-5.78313475674784));
#365639=CARTESIAN_POINT('Ctrl Pts',(-2.02296183383779,-0.0484472105373294,
-5.84358948295386));
#365640=CARTESIAN_POINT('Ctrl Pts',(-1.96637112555623,0.476765831198343,
-5.904047439314));
#365641=CARTESIAN_POINT('Ctrl Pts',(-1.77585742848654,0.969389026837124,
-5.96436475674784));
#365642=CARTESIAN_POINT('Ctrl Pts',(-1.46470738188879,1.39619267968775,
-6.02481948295386));
#365643=CARTESIAN_POINT('Ctrl Pts',(-1.05331000493186,1.72755870948864,
-6.08527743931403));
#365644=CARTESIAN_POINT('Ctrl Pts',(-0.57025927561896,1.94118238458767,
-6.14559475674781));
#365645=CARTESIAN_POINT('Ctrl Pts',(-0.0484472105373227,2.02296183383776,
-6.20604948295386));
#365646=CARTESIAN_POINT('Ctrl Pts',(0.476765831198343,1.96637112555631,
-6.26650743931404));
#365647=CARTESIAN_POINT('Ctrl Pts',(0.969389026837138,1.77585742848649,
-6.32682475674784));
#365648=CARTESIAN_POINT('Ctrl Pts',(1.39619267968763,1.4647073818887,-6.3872794829538));
#365649=CARTESIAN_POINT('Ctrl Pts',(1.72755870948896,1.05331000493196,-6.4477374393141));
#365650=CARTESIAN_POINT('Ctrl Pts',(1.94118238458724,0.570259275618813,
-6.50805475674775));
#365651=CARTESIAN_POINT('Ctrl Pts',(2.0229618338382,0.0484472105380158,
-6.56850948295382));
#365652=CARTESIAN_POINT('Ctrl Pts',(1.96637112555413,-0.47676583120083,
-6.62896743931409));
#365653=CARTESIAN_POINT('Ctrl Pts',(1.77585742849251,-0.969389026833344,
-6.68928475674954));
#365654=CARTESIAN_POINT('Ctrl Pts',(1.46470738188697,-1.39619267969199,
-6.74973948294137));
#365655=CARTESIAN_POINT('Ctrl Pts',(1.05331000488233,-1.72755870945149,
-6.81019743932769));
#365656=CARTESIAN_POINT('Ctrl Pts',(0.570259275809968,-1.94118238475938,
-6.87051475683913));
#365657=CARTESIAN_POINT('Ctrl Pts',(0.0484472101488399,-2.02296183330866,
-6.93096948236246));
#365658=CARTESIAN_POINT('Ctrl Pts',(-0.476765830732716,-1.96637112538019,
-6.99142743997978));
#365659=CARTESIAN_POINT('Ctrl Pts',(-0.969389027651612,-1.775857433288,
-7.05174475889683));
#365660=CARTESIAN_POINT('Ctrl Pts',(-1.39619267380615,-1.46470736293583,
-7.11219946872276));
#365661=CARTESIAN_POINT('Ctrl Pts',(-1.72755871231312,-1.05331002647757,
-7.1726574556236));
#365662=CARTESIAN_POINT('Ctrl Pts',(-1.94118244199894,-0.570259298778077,
-7.23297479041701));
#365663=CARTESIAN_POINT('Ctrl Pts',(-2.02296149561613,-0.0484470734163606,
-7.29342924947211));
#365664=CARTESIAN_POINT('Ctrl Pts',(-1.96637162260829,0.47676563992917,
-7.35388770608518));
#365665=CARTESIAN_POINT('Ctrl Pts',(-1.77585778550465,0.969389377563547,
-7.41420515419699));
#365666=CARTESIAN_POINT('Ctrl Pts',(-1.46470321414872,1.39619055347437,
-7.4746566054593));
#365667=CARTESIAN_POINT('Ctrl Pts',(-1.05331679189158,1.72756279918536,
-7.53512091909894));
#365668=CARTESIAN_POINT('Ctrl Pts',(-0.570256351317271,1.94118541096824,
-7.5954368568002));
#365669=CARTESIAN_POINT('Ctrl Pts',(-0.0484373346474795,2.02291433148142,
-7.65586848775589));
#365670=CARTESIAN_POINT('Ctrl Pts',(0.476753357889169,1.96647633924905,
-7.7163654145941));
#365671=CARTESIAN_POINT('Ctrl Pts',(0.969439733353148,1.77572407380791,
-7.7767079034587));
#365672=CARTESIAN_POINT('Ctrl Pts',(1.39587962475789,1.46484458461224,-7.83687735653918));
#365673=CARTESIAN_POINT('Ctrl Pts',(1.72854436163452,1.05253719801599,-7.89821617217114));
#365674=CARTESIAN_POINT('Ctrl Pts',(1.93848294702123,0.574209674581668,
-7.95584767975511));
#365675=CARTESIAN_POINT('Ctrl Pts',(1.99983638908382,0.21585245779268,-8.0021551741418));
#365676=CARTESIAN_POINT('Ctrl Pts',(1.99983638908381,0.0349322317806574,
-8.0195498399348));
#365677=CARTESIAN_POINT('Ctrl Pts',(2.79994858862227,0.0349509159166703,
-2.22036092810323));
#365678=CARTESIAN_POINT('Ctrl Pts',(2.79994858862227,-0.139575668868676,
-2.2371408740565));
#365679=CARTESIAN_POINT('Ctrl Pts',(2.75037827604958,-0.709564393345761,
-2.28015525707901));
#365680=CARTESIAN_POINT('Ctrl Pts',(2.47621731633814,-1.36758720768895,
-2.33996510409957));
#365681=CARTESIAN_POINT('Ctrl Pts',(2.03652735787686,-1.97060513145091,
-2.40041011005543));
#365682=CARTESIAN_POINT('Ctrl Pts',(1.45882535636765,-2.42725879682614,
-2.46061860312929));
#365683=CARTESIAN_POINT('Ctrl Pts',(0.778984051215511,-2.72322518705085,
-2.52138622529428));
#365684=CARTESIAN_POINT('Ctrl Pts',(0.0484297642119496,-2.83200556197398,
-2.58159582044269));
#365685=CARTESIAN_POINT('Ctrl Pts',(-0.685450641971131,-2.74825639207482,
-2.64190405674164));
#365686=CARTESIAN_POINT('Ctrl Pts',(-1.37463426946475,-2.47632736314912,
-2.70257334387197));
#365687=CARTESIAN_POINT('Ctrl Pts',(-1.96827598629794,-2.03682795409175,
-2.76284677121916));
#365688=CARTESIAN_POINT('Ctrl Pts',(-2.42800955174095,-1.45859372951871,
-2.82313499374427));
#365689=CARTESIAN_POINT('Ctrl Pts',(-2.72304123415184,-0.779023759534372,
-2.88379861057494));
#365690=CARTESIAN_POINT('Ctrl Pts',(-2.8320336979111,-0.048473869777412,
-2.94407960146198));
#365691=CARTESIAN_POINT('Ctrl Pts',(-2.74824361925341,0.685481463726674,
-3.00436484069483));
#365692=CARTESIAN_POINT('Ctrl Pts',(-2.47633436627399,1.37462777686922,
-3.06502821143375));
#365693=CARTESIAN_POINT('Ctrl Pts',(-2.03682617231757,1.96827391913905,
-3.1253098639868));
#365694=CARTESIAN_POINT('Ctrl Pts',(-1.45859315078841,2.42801028311372,
-3.18559480989526));
#365695=CARTESIAN_POINT('Ctrl Pts',(-0.779024215181206,2.72304148177415,
-3.24625818880055));
#365696=CARTESIAN_POINT('Ctrl Pts',(-0.048473746111519,2.83203341149851,
-3.30653988107861));
#365697=CARTESIAN_POINT('Ctrl Pts',(0.685481418057947,2.74824364736727,
-3.36682480706082));
#365698=CARTESIAN_POINT('Ctrl Pts',(1.37462779502025,2.47633440409695,-3.42748818802511));
#365699=CARTESIAN_POINT('Ctrl Pts',(1.96827391500616,2.03682614262167,-3.48776988183974));
#365700=CARTESIAN_POINT('Ctrl Pts',(2.42801027811778,1.45859316111554,-3.54805480689131));
#365701=CARTESIAN_POINT('Ctrl Pts',(2.72304148527533,0.779024213981512,
-3.60871818802593));
#365702=CARTESIAN_POINT('Ctrl Pts',(2.83203341001962,0.0484737449867304,
-3.66899988185579));
#365703=CARTESIAN_POINT('Ctrl Pts',(2.74824364768127,-0.685481417196696,
-3.72928480688587));
#365704=CARTESIAN_POINT('Ctrl Pts',(2.47633440410028,-1.37462779528777,
-3.78994818802735));
#365705=CARTESIAN_POINT('Ctrl Pts',(2.03682614256268,-1.96827391497919,
-3.85022988185542));
#365706=CARTESIAN_POINT('Ctrl Pts',(1.45859316115093,-2.42801027810626,
-3.91051480688602));
#365707=CARTESIAN_POINT('Ctrl Pts',(0.779024213969054,-2.72304148528015,
-3.97117818802726));
#365708=CARTESIAN_POINT('Ctrl Pts',(0.0484737449901392,-2.83203341001849,
-4.03145988185545));
#365709=CARTESIAN_POINT('Ctrl Pts',(-0.685481417197671,-2.74824364768172,
-4.09174480688602));
#365710=CARTESIAN_POINT('Ctrl Pts',(-1.3746277952878,-2.4763344040999,-4.15240818802725));
#365711=CARTESIAN_POINT('Ctrl Pts',(-1.96827391497889,-2.03682614256299,
-4.21268988185546));
#365712=CARTESIAN_POINT('Ctrl Pts',(-2.42801027810644,-1.45859316115073,
-4.27297480688604));
#365713=CARTESIAN_POINT('Ctrl Pts',(-2.72304148528011,-0.779024213969072,
-4.33363818802725));
#365714=CARTESIAN_POINT('Ctrl Pts',(-2.83203341001849,-0.0484737449901639,
-4.39391988185546));
#365715=CARTESIAN_POINT('Ctrl Pts',(-2.7482436476817,0.685481417197704,
-4.45420480688603));
#365716=CARTESIAN_POINT('Ctrl Pts',(-2.4763344040999,1.3746277952878,-4.51486818802725));
#365717=CARTESIAN_POINT('Ctrl Pts',(-2.03682614256298,1.96827391497889,
-4.57514988185546));
#365718=CARTESIAN_POINT('Ctrl Pts',(-1.45859316115072,2.42801027810644,
-4.63543480688604));
#365719=CARTESIAN_POINT('Ctrl Pts',(-0.779024213969067,2.72304148528013,
-4.69609818802723));
#365720=CARTESIAN_POINT('Ctrl Pts',(-0.04847374499015,2.83203341001848,
-4.75637988185547));
#365721=CARTESIAN_POINT('Ctrl Pts',(0.685481417197709,2.7482436476817,-4.81666480688603));
#365722=CARTESIAN_POINT('Ctrl Pts',(1.37462779528781,2.47633440409989,-4.87732818802725));
#365723=CARTESIAN_POINT('Ctrl Pts',(1.9682739149789,2.03682614256298,-4.93760988185546));
#365724=CARTESIAN_POINT('Ctrl Pts',(2.42801027810644,1.4585931611507,-4.99789480688605));
#365725=CARTESIAN_POINT('Ctrl Pts',(2.7230414852801,0.779024213969058,-5.05855818802725));
#365726=CARTESIAN_POINT('Ctrl Pts',(2.83203341001848,0.0484737449901475,
-5.11883988185546));
#365727=CARTESIAN_POINT('Ctrl Pts',(2.74824364768169,-0.685481417197721,
-5.17912480688604));
#365728=CARTESIAN_POINT('Ctrl Pts',(2.47633440409989,-1.37462779528781,
-5.23978818802725));
#365729=CARTESIAN_POINT('Ctrl Pts',(2.03682614256297,-1.9682739149789,-5.30006988185546));
#365730=CARTESIAN_POINT('Ctrl Pts',(1.45859316115069,-2.42801027810645,
-5.36035480688604));
#365731=CARTESIAN_POINT('Ctrl Pts',(0.779024213969056,-2.72304148528011,
-5.42101818802724));
#365732=CARTESIAN_POINT('Ctrl Pts',(0.0484737449901378,-2.83203341001847,
-5.48129988185548));
#365733=CARTESIAN_POINT('Ctrl Pts',(-0.685481417197721,-2.7482436476817,
-5.54158480688602));
#365734=CARTESIAN_POINT('Ctrl Pts',(-1.37462779528784,-2.4763344040999,
-5.60224818802724));
#365735=CARTESIAN_POINT('Ctrl Pts',(-1.9682739149789,-2.03682614256296,
-5.66252988185546));
#365736=CARTESIAN_POINT('Ctrl Pts',(-2.42801027810645,-1.45859316115069,
-5.72281480688604));
#365737=CARTESIAN_POINT('Ctrl Pts',(-2.72304148528013,-0.779024213969052,
-5.78347818802723));
#365738=CARTESIAN_POINT('Ctrl Pts',(-2.83203341001847,-0.0484737449901258,
-5.84375988185547));
#365739=CARTESIAN_POINT('Ctrl Pts',(-2.74824364768167,0.685481417197731,
-5.90404480688604));
#365740=CARTESIAN_POINT('Ctrl Pts',(-2.47633440409989,1.37462779528784,
-5.96470818802724));
#365741=CARTESIAN_POINT('Ctrl Pts',(-2.03682614256295,1.96827391497889,
-6.02498988185547));
#365742=CARTESIAN_POINT('Ctrl Pts',(-1.4585931611507,2.42801027810647,-6.08527480688602));
#365743=CARTESIAN_POINT('Ctrl Pts',(-0.779024213969003,2.7230414852801,
-6.14593818802726));
#365744=CARTESIAN_POINT('Ctrl Pts',(-0.0484737449901475,2.83203341001844,
-6.20621988185547));
#365745=CARTESIAN_POINT('Ctrl Pts',(0.685481417197711,2.74824364768178,
-6.266504806886));
#365746=CARTESIAN_POINT('Ctrl Pts',(1.37462779528805,2.4763344040997,-6.32716818802727));
#365747=CARTESIAN_POINT('Ctrl Pts',(1.96827391497844,2.03682614256313,-6.3874498818555));
#365748=CARTESIAN_POINT('Ctrl Pts',(2.42801027810703,1.45859316115076,-6.44773480688596));
#365749=CARTESIAN_POINT('Ctrl Pts',(2.72304148527948,0.779024213968036,
-6.50839818802743));
#365750=CARTESIAN_POINT('Ctrl Pts',(2.83203341001966,0.0484737449934034,
-6.56867988185514));
#365751=CARTESIAN_POINT('Ctrl Pts',(2.74824364767639,-0.685481417209638,
-6.62896480688735));
#365752=CARTESIAN_POINT('Ctrl Pts',(2.47633440411674,-1.37462779525554,
-6.68962818802195));
#365753=CARTESIAN_POINT('Ctrl Pts',(2.03682614255995,-1.96827391501936,
-6.74990988187118));
#365754=CARTESIAN_POINT('Ctrl Pts',(1.45859316092616,-2.42801027811759,
-6.81019480688936));
#365755=CARTESIAN_POINT('Ctrl Pts',(0.779024214864112,-2.72304148523437,
-6.87085818784773));
#365756=CARTESIAN_POINT('Ctrl Pts',(0.0484737436638102,-2.83203340983582,
-6.93113988263782));
#365757=CARTESIAN_POINT('Ctrl Pts',(-0.685481418136962,-2.74824364633194,
-6.99142480614438));
#365758=CARTESIAN_POINT('Ctrl Pts',(-1.37462778885995,-2.47633441354984,
-7.05208818488281));
#365759=CARTESIAN_POINT('Ctrl Pts',(-1.96827391894949,-2.03682611603706,
-7.11236989989014));
#365760=CARTESIAN_POINT('Ctrl Pts',(-2.42801027659746,-1.45859318121514,
-7.17265478410175));
#365761=CARTESIAN_POINT('Ctrl Pts',(-2.72304154587753,-0.779024258186026,
-7.23331815145116));
#365762=CARTESIAN_POINT('Ctrl Pts',(-2.83203304292954,-0.0484735881915938,
-7.29360016643431));
#365763=CARTESIAN_POINT('Ctrl Pts',(-2.74824426833468,0.685481026990187,
-7.35388438911616));
#365764=CARTESIAN_POINT('Ctrl Pts',(-2.47633426068,1.37462897834074,-7.41454797566736));
#365765=CARTESIAN_POINT('Ctrl Pts',(-2.03682260074525,1.96827080720847,
-7.47483300656648));
#365766=CARTESIAN_POINT('Ctrl Pts',(-1.45860575946508,2.42800983497797,
-7.53510984362855));
#365767=CARTESIAN_POINT('Ctrl Pts',(-0.778993598834234,2.72306539561668,
-7.59577812434582));
#365768=CARTESIAN_POINT('Ctrl Pts',(-0.0485111105849109,2.83192268777547,
-7.65608621916571));
#365769=CARTESIAN_POINT('Ctrl Pts',(0.685434178093518,2.74858121042738,
-7.71629032556075));
#365770=CARTESIAN_POINT('Ctrl Pts',(1.37494905476715,2.47530931106774,-7.77708760315606));
#365771=CARTESIAN_POINT('Ctrl Pts',(1.96749699730902,2.03997328191583,-7.83717861739831));
#365772=CARTESIAN_POINT('Ctrl Pts',(2.42925527357646,1.44798370557448,-7.89806652053729));
#365773=CARTESIAN_POINT('Ctrl Pts',(2.72026578942101,0.81850829674785,-7.95608482081467));
#365774=CARTESIAN_POINT('Ctrl Pts',(2.7998363224979,0.209484955020671,-8.00303038055522));
#365775=CARTESIAN_POINT('Ctrl Pts',(2.7998363224979,0.0349606549170308,
-8.01981010684662));
#365776=CARTESIAN_POINT('Ctrl Pts',(2.80005140479051,-0.0349419760186688,
-1.58036093336367));
#365777=CARTESIAN_POINT('Ctrl Pts',(2.80005140479051,-0.222315492003956,
-1.59837605395503));
#365778=CARTESIAN_POINT('Ctrl Pts',(2.7214217418683,-0.809145725726729,
-1.6432251028271));
#365779=CARTESIAN_POINT('Ctrl Pts',(2.4293855576505,-1.45019120570836,-1.70229805797781));
#365780=CARTESIAN_POINT('Ctrl Pts',(1.96768973634555,-2.03953853811049,
-1.7629395123984));
#365781=CARTESIAN_POINT('Ctrl Pts',(1.37507506915162,-2.47563743577604,
-1.8230967134397));
#365782=CARTESIAN_POINT('Ctrl Pts',(0.685513462117749,-2.74874432479135,
-1.88387667036327));
#365783=CARTESIAN_POINT('Ctrl Pts',(-0.0484811831405424,-2.83215111147164,
-1.94408480572724));
#365784=CARTESIAN_POINT('Ctrl Pts',(-0.779026681647449,-2.72327925825339,
-2.00439212797816));
#365785=CARTESIAN_POINT('Ctrl Pts',(-1.45869410662288,-2.42821024693195,
-2.0650608706179));
#365786=CARTESIAN_POINT('Ctrl Pts',(-2.03695498339253,-1.96844588111817,
-2.12533700840671));
#365787=CARTESIAN_POINT('Ctrl Pts',(-2.4765110806735,-1.3747587008243,-2.18562256240842));
#365788=CARTESIAN_POINT('Ctrl Pts',(-2.7484478409841,-0.685559860459645,
-2.24628623797644));
#365789=CARTESIAN_POINT('Ctrl Pts',(-2.83225060905395,0.048443263325025,
-2.30656987054029));
#365790=CARTESIAN_POINT('Ctrl Pts',(-2.72325825549342,0.779057613295582,
-2.36685238231703));
#365791=CARTESIAN_POINT('Ctrl Pts',(-2.42820998732486,1.45868136138043,
-2.4275158429718));
#365792=CARTESIAN_POINT('Ctrl Pts',(-1.96844920055485,2.03695852016992,
-2.48780013698524));
#365793=CARTESIAN_POINT('Ctrl Pts',(-1.37475744002027,2.4765112353038,-2.54808234902813));
#365794=CARTESIAN_POINT('Ctrl Pts',(-0.685560283084277,2.74844721593019,
-2.60874582079915));
#365795=CARTESIAN_POINT('Ctrl Pts',(0.0484434248256224,2.83225097648717,
-2.66903015426646));
#365796=CARTESIAN_POINT('Ctrl Pts',(0.7790575695397,2.72325819429533,-2.72931234606168));
#365797=CARTESIAN_POINT('Ctrl Pts',(1.45868134037711,2.42820998953338,-2.78997582004938));
#365798=CARTESIAN_POINT('Ctrl Pts',(2.0369585467678,1.96844919652417,-2.85026015503416));
#365799=CARTESIAN_POINT('Ctrl Pts',(2.47651122587901,1.37475744638445,-2.91054234588739));
#365800=CARTESIAN_POINT('Ctrl Pts',(2.74844721726047,0.68556028222042,-2.97120582005121));
#365801=CARTESIAN_POINT('Ctrl Pts',(2.8322509766735,-0.0484434261664062,
-3.03149015505023));
#365802=CARTESIAN_POINT('Ctrl Pts',(2.7232581943391,-0.779057568642653,
-3.09177234588191));
#365803=CARTESIAN_POINT('Ctrl Pts',(2.42820998952435,-1.45868134060022,
-3.15243582005264));
#365804=CARTESIAN_POINT('Ctrl Pts',(1.9684491964829,-2.03695854677124,-3.21272015504985));
#365805=CARTESIAN_POINT('Ctrl Pts',(1.37475744641701,-2.4765112258619,-3.27300234588205));
#365806=CARTESIAN_POINT('Ctrl Pts',(0.685560282208511,-2.74844721726587,
-3.33366582005255));
#365807=CARTESIAN_POINT('Ctrl Pts',(-0.0484434261631521,-2.83225097667228,
-3.39395015504989));
#365808=CARTESIAN_POINT('Ctrl Pts',(-0.779057568643627,-2.7232581943397,
-3.45423234588206));
#365809=CARTESIAN_POINT('Ctrl Pts',(-1.45868134060013,-2.42820998952376,
-3.51489582005254));
#365810=CARTESIAN_POINT('Ctrl Pts',(-2.03695854677107,-1.96844919648335,
-3.57518015504989));
#365811=CARTESIAN_POINT('Ctrl Pts',(-2.47651122586207,-1.3747574464168,
-3.63546234588207));
#365812=CARTESIAN_POINT('Ctrl Pts',(-2.74844721726579,-0.685560282208525,
-3.69612582005254));
#365813=CARTESIAN_POINT('Ctrl Pts',(-2.83225097667231,0.0484434261631291,
-3.7564101550499));
#365814=CARTESIAN_POINT('Ctrl Pts',(-2.7232581943397,0.779057568643663,
-3.81669234588207));
#365815=CARTESIAN_POINT('Ctrl Pts',(-2.42820998952376,1.45868134060013,
-3.87735582005254));
#365816=CARTESIAN_POINT('Ctrl Pts',(-1.96844919648335,2.03695854677107,
-3.9376401550499));
#365817=CARTESIAN_POINT('Ctrl Pts',(-1.37475744641679,2.47651122586208,
-3.99792234588207));
#365818=CARTESIAN_POINT('Ctrl Pts',(-0.685560282208515,2.74844721726578,
-4.05858582005252));
#365819=CARTESIAN_POINT('Ctrl Pts',(0.0484434261631405,2.83225097667232,
-4.1188701550499));
#365820=CARTESIAN_POINT('Ctrl Pts',(0.779057568643667,2.72325819433969,
-4.17915234588206));
#365821=CARTESIAN_POINT('Ctrl Pts',(1.45868134060014,2.42820998952375,-4.23981582005254));
#365822=CARTESIAN_POINT('Ctrl Pts',(2.03695854677108,1.96844919648334,-4.30010015504989));
#365823=CARTESIAN_POINT('Ctrl Pts',(2.47651122586209,1.37475744641679,-4.36038234588208));
#365824=CARTESIAN_POINT('Ctrl Pts',(2.74844721726579,0.685560282208506,
-4.42104582005254));
#365825=CARTESIAN_POINT('Ctrl Pts',(2.8322509766723,-0.0484434261631421,
-4.4813301550499));
#365826=CARTESIAN_POINT('Ctrl Pts',(2.72325819433969,-0.779057568643682,
-4.54161234588207));
#365827=CARTESIAN_POINT('Ctrl Pts',(2.42820998952373,-1.45868134060014,
-4.60227582005254));
#365828=CARTESIAN_POINT('Ctrl Pts',(1.96844919648334,-2.03695854677108,
-4.6625601550499));
#365829=CARTESIAN_POINT('Ctrl Pts',(1.37475744641678,-2.47651122586209,
-4.72284234588207));
#365830=CARTESIAN_POINT('Ctrl Pts',(0.685560282208503,-2.74844721726579,
-4.78350582005254));
#365831=CARTESIAN_POINT('Ctrl Pts',(-0.0484434261631558,-2.83225097667233,
-4.84379015504992));
#365832=CARTESIAN_POINT('Ctrl Pts',(-0.77905756864368,-2.72325819433967,
-4.90407234588205));
#365833=CARTESIAN_POINT('Ctrl Pts',(-1.45868134060014,-2.42820998952372,
-4.96473582005253));
#365834=CARTESIAN_POINT('Ctrl Pts',(-2.03695854677109,-1.96844919648334,
-5.0250201550499));
#365835=CARTESIAN_POINT('Ctrl Pts',(-2.47651122586209,-1.37475744641677,
-5.08530234588207));
#365836=CARTESIAN_POINT('Ctrl Pts',(-2.74844721726577,-0.685560282208494,
-5.14596582005252));
#365837=CARTESIAN_POINT('Ctrl Pts',(-2.83225097667232,0.0484434261631642,
-5.20625015504991));
#365838=CARTESIAN_POINT('Ctrl Pts',(-2.72325819433969,0.779057568643699,
-5.26653234588207));
#365839=CARTESIAN_POINT('Ctrl Pts',(-2.42820998952371,1.45868134060015,
-5.32719582005253));
#365840=CARTESIAN_POINT('Ctrl Pts',(-1.96844919648334,2.0369585467711,-5.38748015504991));
#365841=CARTESIAN_POINT('Ctrl Pts',(-1.37475744641676,2.47651122586207,
-5.44776234588206));
#365842=CARTESIAN_POINT('Ctrl Pts',(-0.685560282208465,2.74844721726582,
-5.50842582005256));
#365843=CARTESIAN_POINT('Ctrl Pts',(0.0484434261631459,2.8322509766723,
-5.56871015504991));
#365844=CARTESIAN_POINT('Ctrl Pts',(0.77905756864366,2.7232581943397,-5.62899234588203));
#365845=CARTESIAN_POINT('Ctrl Pts',(1.45868134060035,2.42820998952354,-5.68965582005256));
#365846=CARTESIAN_POINT('Ctrl Pts',(2.03695854677077,1.96844919648363,-5.74994015504994));
#365847=CARTESIAN_POINT('Ctrl Pts',(2.47651122586247,1.37475744641675,-5.81022234588199));
#365848=CARTESIAN_POINT('Ctrl Pts',(2.74844721726539,0.68556028220749,-5.87088582005272));
#365849=CARTESIAN_POINT('Ctrl Pts',(2.83225097667343,-0.0484434261597295,
-5.93117015504957));
#365850=CARTESIAN_POINT('Ctrl Pts',(2.72325819433488,-0.779057568656138,
-5.99145234588337));
#365851=CARTESIAN_POINT('Ctrl Pts',(2.42820998953502,-1.45868134056502,
-6.05211582004729));
#365852=CARTESIAN_POINT('Ctrl Pts',(1.96844919651089,-2.03695854682948,
-6.11240015506561));
#365853=CARTESIAN_POINT('Ctrl Pts',(1.37475744614754,-2.47651122586056,
-6.17268234588436));
#365854=CARTESIAN_POINT('Ctrl Pts',(0.685560283068197,-2.7484472169499,
-6.2333458198777));
#365855=CARTESIAN_POINT('Ctrl Pts',(-0.0484434272739145,-2.83225097815536,
-6.29363015582641));
#365856=CARTESIAN_POINT('Ctrl Pts',(-0.779057569919619,-2.72325819081683,
-6.35391234511296));
#365857=CARTESIAN_POINT('Ctrl Pts',(-1.45868133020244,-2.42820999454269,
-6.41457581704206));
#365858=CARTESIAN_POINT('Ctrl Pts',(-2.03695857643473,-1.96844920071866,
-6.47486017290601));
#365859=CARTESIAN_POINT('Ctrl Pts',(-2.47651118869187,-1.37475742725566,
-6.53514232258922));
#365860=CARTESIAN_POINT('Ctrl Pts',(-2.74844718829262,-0.685560328345768,
-6.59580578606602));
#365861=CARTESIAN_POINT('Ctrl Pts',(-2.83225126519656,0.0484435449931018,
-6.65609043578674));
#365862=CARTESIAN_POINT('Ctrl Pts',(-2.72325793947389,0.779057145346554,
-6.71637192313681));
#365863=CARTESIAN_POINT('Ctrl Pts',(-2.42820926584284,1.45868183876673,
-6.77703563697173));
#365864=CARTESIAN_POINT('Ctrl Pts',(-1.9684512872418,2.03696056375976,-6.83732324720959));
#365865=CARTESIAN_POINT('Ctrl Pts',(-1.37476376271817,2.47650348514813,
-6.89759727195412));
#365866=CARTESIAN_POINT('Ctrl Pts',(-0.685529731491166,2.74846279478609,
-6.95826629062831));
#365867=CARTESIAN_POINT('Ctrl Pts',(0.0483996833656258,2.8322123503721,
-7.01857521801487));
#365868=CARTESIAN_POINT('Ctrl Pts',(0.779017444894231,2.72348202273134,
-7.07878068295039));
#365869=CARTESIAN_POINT('Ctrl Pts',(1.45891552110071,2.42730834706515,-7.13956566066343));
#365870=CARTESIAN_POINT('Ctrl Pts',(2.03664883326185,1.97134324740292,-7.19970870776557));
#365871=CARTESIAN_POINT('Ctrl Pts',(2.47643830365019,1.36561422989075,-7.2603969994144));
#365872=CARTESIAN_POINT('Ctrl Pts',(2.74977893008757,0.719015851050413,
-7.31916157554443));
#365873=CARTESIAN_POINT('Ctrl Pts',(2.80016361091614,0.126800216505963,
-7.36426031277698));
#365874=CARTESIAN_POINT('Ctrl Pts',(2.80016361091613,-0.0349322317809129,
-7.37981016006518));
#365875=CARTESIAN_POINT('Ctrl Pts',(2.00005141137773,-0.0349509159166537,
-1.58027907189674));
#365876=CARTESIAN_POINT('Ctrl Pts',(2.00005141137773,-0.209477500702,-1.59705901785001));
#365877=CARTESIAN_POINT('Ctrl Pts',(1.93937485936534,-0.574981221086946,
-1.64398167301615));
#365878=CARTESIAN_POINT('Ctrl Pts',(1.72866575619624,-1.05218683017129,
-1.70157781695483));
#365879=CARTESIAN_POINT('Ctrl Pts',(1.39603065320521,-1.46514475575449,
-1.76296158741006));
#365880=CARTESIAN_POINT('Ctrl Pts',(0.969522180315677,-1.77589106055163,
-1.82311912419573));
#365881=CARTESIAN_POINT('Ctrl Pts',(0.476783238604109,-1.96670288995313,
-1.88346520364747));
#365882=CARTESIAN_POINT('Ctrl Pts',(-0.0484603850821368,-2.02312932285366,
-1.94396055370022));
#365883=CARTESIAN_POINT('Ctrl Pts',(-0.570338856925993,-1.94138942628423,
-2.00439291407465));
#365884=CARTESIAN_POINT('Ctrl Pts',(-1.05344948325284,-1.72773686772633,
-2.06470891120488));
#365885=CARTESIAN_POINT('Ctrl Pts',(-1.46487312544728,-1.39632835696345,
-2.1251726344757));
#365886=CARTESIAN_POINT('Ctrl Pts',(-1.77606001340043,-0.969474639293403,
-2.18562457894241));
#365887=CARTESIAN_POINT('Ctrl Pts',(-1.9665886161183,-0.476795144252666,
-2.2459421237894));
#365888=CARTESIAN_POINT('Ctrl Pts',(-2.0231790616074,0.0484698229690482,
-2.30639998925771));
#365889=CARTESIAN_POINT('Ctrl Pts',(-1.94138573006516,0.570342005097921,
-2.36685494461854));
#365890=CARTESIAN_POINT('Ctrl Pts',(-1.72773301625381,1.05344259449438,
-2.42717237256682));
#365891=CARTESIAN_POINT('Ctrl Pts',(-1.39633042998923,1.46487729238585,
-2.48762977035772));
#365892=CARTESIAN_POINT('Ctrl Pts',(-0.969474291036093,1.77605966206198,
-2.54808497616048));
#365893=CARTESIAN_POINT('Ctrl Pts',(-0.476795343347378,1.96658811640277,
-2.6084023881129));
#365894=CARTESIAN_POINT('Ctrl Pts',(0.0484699602192744,2.02317939996145,
-2.66885975673847));
#365895=CARTESIAN_POINT('Ctrl Pts',(0.570341982836039,1.94138567238666,
-2.72931497821885));
#365896=CARTESIAN_POINT('Ctrl Pts',(1.05344257210098,1.72773301387229,-2.78963238875962));
#365897=CARTESIAN_POINT('Ctrl Pts',(1.46487731147791,1.39633043581364,-2.85008975616076));
#365898=CARTESIAN_POINT('Ctrl Pts',(1.7760596572503,0.96947429019414,-2.91054497830833));
#365899=CARTESIAN_POINT('Ctrl Pts',(1.96658811657123,0.47679534386094,-2.97086238877306));
#365900=CARTESIAN_POINT('Ctrl Pts',(2.02317940049204,-0.0484699606166185,
-3.03131975614836));
#365901=CARTESIAN_POINT('Ctrl Pts',(1.94138567221384,-0.570341982644115,
-3.09177497831011));
#365902=CARTESIAN_POINT('Ctrl Pts',(1.72773301391076,-1.05344257214956,
-3.15209238877301));
#365903=CARTESIAN_POINT('Ctrl Pts',(1.39633043580907,-1.46487731147983,
-3.21254975614839));
#365904=CARTESIAN_POINT('Ctrl Pts',(0.969474290197969,-1.77605965724421,
-3.27300497831004));
#365905=CARTESIAN_POINT('Ctrl Pts',(0.476795343858464,-1.96658811657341,
-3.33332238877311));
#365906=CARTESIAN_POINT('Ctrl Pts',(-0.0484699606159255,-2.0231794004916,
-3.39377975614832));
#365907=CARTESIAN_POINT('Ctrl Pts',(-0.570341982644268,-1.94138567221424,
-3.45423497831005));
#365908=CARTESIAN_POINT('Ctrl Pts',(-1.05344257214943,-1.72773301391041,
-3.51455238877311));
#365909=CARTESIAN_POINT('Ctrl Pts',(-1.46487731147993,-1.39633043580919,
-3.57500975614831));
#365910=CARTESIAN_POINT('Ctrl Pts',(-1.77605965724425,-0.969474290197954,
-3.63546497831004));
#365911=CARTESIAN_POINT('Ctrl Pts',(-1.96658811657337,-0.476795343858458,
-3.69578238877312));
#365912=CARTESIAN_POINT('Ctrl Pts',(-2.02317940049162,0.0484699606159343,
-3.75623975614831));
#365913=CARTESIAN_POINT('Ctrl Pts',(-1.94138567221425,0.570341982644281,
-3.81669497831005));
#365914=CARTESIAN_POINT('Ctrl Pts',(-1.7277330139104,1.05344257214943,-3.87701238877311));
#365915=CARTESIAN_POINT('Ctrl Pts',(-1.39633043580919,1.46487731147993,
-3.93746975614831));
#365916=CARTESIAN_POINT('Ctrl Pts',(-0.969474290197942,1.77605965724426,
-3.99792497831004));
#365917=CARTESIAN_POINT('Ctrl Pts',(-0.476795343858452,1.96658811657335,
-4.05824238877313));
#365918=CARTESIAN_POINT('Ctrl Pts',(0.0484699606159434,2.02317940049163,
-4.11869975614831));
#365919=CARTESIAN_POINT('Ctrl Pts',(0.570341982644284,1.94138567221424,
-4.17915497831005));
#365920=CARTESIAN_POINT('Ctrl Pts',(1.05344257214943,1.72773301391039,-4.23947238877311));
#365921=CARTESIAN_POINT('Ctrl Pts',(1.46487731147993,1.39633043580918,-4.29992975614832));
#365922=CARTESIAN_POINT('Ctrl Pts',(1.77605965724427,0.969474290197945,
-4.36038497831003));
#365923=CARTESIAN_POINT('Ctrl Pts',(1.96658811657337,0.476795343858441,
-4.42070238877312));
#365924=CARTESIAN_POINT('Ctrl Pts',(2.02317940049162,-0.0484699606159445,
-4.48115975614831));
#365925=CARTESIAN_POINT('Ctrl Pts',(1.94138567221424,-0.570341982644292,
-4.54161497831005));
#365926=CARTESIAN_POINT('Ctrl Pts',(1.72773301391038,-1.05344257214943,
-4.60193238877312));
#365927=CARTESIAN_POINT('Ctrl Pts',(1.39633043580918,-1.46487731147994,
-4.66238975614831));
#365928=CARTESIAN_POINT('Ctrl Pts',(0.969474290197935,-1.77605965724426,
-4.72284497831004));
#365929=CARTESIAN_POINT('Ctrl Pts',(0.476795343858439,-1.96658811657337,
-4.78316238877312));
#365930=CARTESIAN_POINT('Ctrl Pts',(-0.0484699606159579,-2.02317940049164,
-4.8436197561483));
#365931=CARTESIAN_POINT('Ctrl Pts',(-0.570341982644288,-1.94138567221422,
-4.90407497831006));
#365932=CARTESIAN_POINT('Ctrl Pts',(-1.05344257214943,-1.72773301391037,
-4.96439238877312));
#365933=CARTESIAN_POINT('Ctrl Pts',(-1.46487731147995,-1.39633043580918,
-5.02484975614831));
#365934=CARTESIAN_POINT('Ctrl Pts',(-1.77605965724426,-0.969474290197928,
-5.08530497831004));
#365935=CARTESIAN_POINT('Ctrl Pts',(-1.96658811657335,-0.476795343858433,
-5.14562238877313));
#365936=CARTESIAN_POINT('Ctrl Pts',(-2.02317940049163,0.0484699606159606,
-5.2060797561483));
#365937=CARTESIAN_POINT('Ctrl Pts',(-1.94138567221425,0.570341982644311,
-5.26653497831003));
#365938=CARTESIAN_POINT('Ctrl Pts',(-1.72773301391036,1.05344257214944,
-5.32685238877313));
#365939=CARTESIAN_POINT('Ctrl Pts',(-1.39633043580918,1.46487731147996,
-5.3873097561483));
#365940=CARTESIAN_POINT('Ctrl Pts',(-0.969474290197916,1.77605965724424,
-5.44776497831006));
#365941=CARTESIAN_POINT('Ctrl Pts',(-0.476795343858422,1.96658811657339,
-5.5080823887731));
#365942=CARTESIAN_POINT('Ctrl Pts',(0.0484699606159706,2.02317940049163,
-5.56853975614829));
#365943=CARTESIAN_POINT('Ctrl Pts',(0.570341982644291,1.94138567221422,
-5.62899497831007));
#365944=CARTESIAN_POINT('Ctrl Pts',(1.05344257214944,1.72773301391032,-5.68931238877313));
#365945=CARTESIAN_POINT('Ctrl Pts',(1.46487731147996,1.3963304358092,-5.74976975614823));
#365946=CARTESIAN_POINT('Ctrl Pts',(1.77605965724441,0.969474290197947,
-5.81022497831013));
#365947=CARTESIAN_POINT('Ctrl Pts',(1.96658811657315,0.476795343858267,
-5.87054238877304));
#365948=CARTESIAN_POINT('Ctrl Pts',(2.02317940049197,-0.0484699606151168,
-5.93099975614826));
#365949=CARTESIAN_POINT('Ctrl Pts',(1.94138567221262,-0.570341982647331,
-5.99145497831012));
#365950=CARTESIAN_POINT('Ctrl Pts',(1.72773301391079,-1.05344257214282,
-6.05177238877488));
#365951=CARTESIAN_POINT('Ctrl Pts',(1.39633043583791,-1.46487731150212,
-6.1122297561358));
#365952=CARTESIAN_POINT('Ctrl Pts',(0.969474290103704,-1.77605965719443,
-6.17268497832268));
#365953=CARTESIAN_POINT('Ctrl Pts',(0.476795344014053,-1.96658811647506,
-6.23300238886911));
#365954=CARTESIAN_POINT('Ctrl Pts',(-0.0484699607888847,-2.02317940162764,
-6.293459755551));
#365955=CARTESIAN_POINT('Ctrl Pts',(-0.570341982515374,-1.94138566986718,
-6.35391497894857));
#365956=CARTESIAN_POINT('Ctrl Pts',(-1.0534425689941,-1.72773301427299,
-6.41423239105532));
#365957=CARTESIAN_POINT('Ctrl Pts',(-1.46487733129139,-1.39633044764682,
-6.47468974174144));
#365958=CARTESIAN_POINT('Ctrl Pts',(-1.77605962440754,-0.969474272408487,
-6.53514499410053));
#365959=CARTESIAN_POINT('Ctrl Pts',(-1.96658808441403,-0.4767953693466,
-6.59546242507117));
#365960=CARTESIAN_POINT('Ctrl Pts',(-2.02317971788315,0.0484700612956726,
-6.65591951867769));
#365961=CARTESIAN_POINT('Ctrl Pts',(-1.94138529374751,0.57034175258804,
-6.71637524065362));
#365962=CARTESIAN_POINT('Ctrl Pts',(-1.7277327906675,1.05344225923825,-6.77669281345839));
#365963=CARTESIAN_POINT('Ctrl Pts',(-1.39633190064527,1.46488023063332,
-6.83714685373563));
#365964=CARTESIAN_POINT('Ctrl Pts',(-0.969474795144666,1.77605674551469,
-6.89760831895014));
#365965=CARTESIAN_POINT('Ctrl Pts',(-0.476792483974202,1.96658170561334,
-6.95792512927773));
#365966=CARTESIAN_POINT('Ctrl Pts',(0.0484734593030573,2.0232081210323,
-7.01835708981697));
#365967=CARTESIAN_POINT('Ctrl Pts',(0.570336624689882,1.94136175768686,
-7.07885725203471));
#365968=CARTESIAN_POINT('Ctrl Pts',(1.05340619968671,1.72778052727257,-7.13918044053492));
#365969=CARTESIAN_POINT('Ctrl Pts',(1.46503146071072,1.39600002911185,-7.19942807213429));
#365970=CARTESIAN_POINT('Ctrl Pts',(1.77572739170825,0.970967789756964,
-7.26046972816476));
#365971=CARTESIAN_POINT('Ctrl Pts',(1.9679960876878,0.471734127632586,-7.31921124624962));
#365972=CARTESIAN_POINT('Ctrl Pts',(2.00016367750205,0.139563645186354,
-7.36277016686196));
#365973=CARTESIAN_POINT('Ctrl Pts',(2.00016367750204,-0.0349606549172864,
-7.37954989315336));
#365974=CARTESIAN_POINT('',(2.40000003347425,-1.4296958965801E-5,-7.69954908463262));
#365975=CARTESIAN_POINT('Origin',(2.00000003329294,-1.42115683144641E-5,
-7.69954986654408));
#365976=CARTESIAN_POINT('Origin',(2.00000003329294,-1.42115683144641E-5,
-7.69954986654408));
#365977=CARTESIAN_POINT('Origin',(1.99978500519318,0.0219216792995357,-8.68039848401339));
#365978=CARTESIAN_POINT('Origin',(2.00000005748081,-1.17200745147024E-5,
-8.35982870408561));
#365979=CARTESIAN_POINT('Ctrl Pts',(2.00016367750204,-0.0349606549171534,
-7.37954989315335));
#365980=CARTESIAN_POINT('Ctrl Pts',(2.00016367750204,-0.165462727384539,
-7.38526442622049));
#365981=CARTESIAN_POINT('Ctrl Pts',(1.96855967425598,-0.409173319918984,
-7.39995586097472));
#365982=CARTESIAN_POINT('Ctrl Pts',(1.85189486927969,-0.792213245836797,
-7.42009815347362));
#365983=CARTESIAN_POINT('Ctrl Pts',(1.6613582879716,-1.13645205609876,-7.44086906835104));
#365984=CARTESIAN_POINT('Ctrl Pts',(1.37992038202068,-1.47263550497672,
-7.46380724865708));
#365985=CARTESIAN_POINT('Ctrl Pts',(0.992206889613594,-1.76297069041634,
-7.48903838801854));
#365986=CARTESIAN_POINT('Ctrl Pts',(0.502190643379444,-1.95990154002328,
-7.51648926813145));
#365987=CARTESIAN_POINT('Ctrl Pts',(-0.0222096198383131,-2.0232383143754,
-7.54405136994835));
#365988=CARTESIAN_POINT('Ctrl Pts',(-0.545023222850085,-1.94828998299833,
-7.57157271170469));
#365989=CARTESIAN_POINT('Ctrl Pts',(-1.0307284358197,-1.74090605654878,
-7.59904290948243));
#365990=CARTESIAN_POINT('Ctrl Pts',(-1.44636321247892,-1.41496070139146,
-7.62658089390187));
#365991=CARTESIAN_POINT('Ctrl Pts',(-1.7630429012686,-0.992255621812916,
-7.65411407831587));
#365992=CARTESIAN_POINT('Ctrl Pts',(-1.95983623864864,-0.502172632985278,
-7.68158430816739));
#365993=CARTESIAN_POINT('Ctrl Pts',(-2.02326404614228,0.0222054813197516,
-7.70911956348259));
#365994=CARTESIAN_POINT('Ctrl Pts',(-1.94828990091774,0.545028935894718,
-7.73665436795491));
#365995=CARTESIAN_POINT('Ctrl Pts',(-1.74090287629493,1.03072354235614,
-7.76412460420479));
#365996=CARTESIAN_POINT('Ctrl Pts',(-1.41496257868532,1.44636639725859,
-7.79165822650409));
#365997=CARTESIAN_POINT('Ctrl Pts',(-0.992256976006747,1.76304240583952,
-7.81919574931953));
#365998=CARTESIAN_POINT('Ctrl Pts',(-0.502167983314945,1.95983220557862,
-7.84666606566923));
#365999=CARTESIAN_POINT('Ctrl Pts',(0.0222021542767409,2.02327125956959,
-7.87418752174917));
#366000=CARTESIAN_POINT('Ctrl Pts',(0.545036582780956,1.94830483935279,
-7.90174989061211));
#366001=CARTESIAN_POINT('Ctrl Pts',(1.03068639649234,1.74088018296961,-7.92919874059292));
#366002=CARTESIAN_POINT('Ctrl Pts',(1.41193217216583,1.44192597876132,-7.95443773023923));
#366003=CARTESIAN_POINT('Ctrl Pts',(1.68594383364152,1.10008635709056,-7.97735256352204));
#366004=CARTESIAN_POINT('Ctrl Pts',(1.86832284879594,0.749865410246654,
-7.99820416287286));
#366005=CARTESIAN_POINT('Ctrl Pts',(1.97885834740452,0.370827498858678,
-8.01808024799317));
#366006=CARTESIAN_POINT('Ctrl Pts',(2.00021510976845,0.108553308485772,
-8.03354455068052));
#366007=CARTESIAN_POINT('Ctrl Pts',(2.00021510976845,-0.0219451194485651,
-8.03925892415782));
#366008=CARTESIAN_POINT('Ctrl Pts',(2.80016361091613,-0.03493223178078,
-7.37981016006517));
#366009=CARTESIAN_POINT('Ctrl Pts',(2.80016361091613,-0.178346676400516,
-7.38609011080151));
#366010=CARTESIAN_POINT('Ctrl Pts',(2.75800714240104,-0.585623740854942,
-7.39993625174015));
#366011=CARTESIAN_POINT('Ctrl Pts',(2.59622001092688,-1.094203255455,-7.42050939398873));
#366012=CARTESIAN_POINT('Ctrl Pts',(2.33073889442298,-1.58539648585596,
-7.44121574714249));
#366013=CARTESIAN_POINT('Ctrl Pts',(1.93774673958377,-2.05527341692013,
-7.46406250879474));
#366014=CARTESIAN_POINT('Ctrl Pts',(1.3977924816811,-2.46335493607239,-7.4892382031805));
#366015=CARTESIAN_POINT('Ctrl Pts',(0.710887177607718,-2.74177962175189,
-7.51690579573811));
#366016=CARTESIAN_POINT('Ctrl Pts',(-0.0222315527777081,-2.83230238724503,
-7.54433060281804));
#366017=CARTESIAN_POINT('Ctrl Pts',(-0.753696284786715,-2.73017360349673,
-7.57179577476958));
#366018=CARTESIAN_POINT('Ctrl Pts',(-1.4359964022639,-2.44137112409355,
-7.59942818098223));
#366019=CARTESIAN_POINT('Ctrl Pts',(-2.01844596000972,-1.98707136838064,
-7.62687978029761));
#366020=CARTESIAN_POINT('Ctrl Pts',(-2.46348770759376,-1.39755415476222,
-7.65433629789662));
#366021=CARTESIAN_POINT('Ctrl Pts',(-2.74170364490091,-0.710913395495067,
-7.6819659616779));
#366022=CARTESIAN_POINT('Ctrl Pts',(-2.83233201369082,0.0221843029796173,
-7.70942122438771));
#366023=CARTESIAN_POINT('Ctrl Pts',(-2.73016814474818,0.753729685089645,
-7.73687603703565));
#366024=CARTESIAN_POINT('Ctrl Pts',(-2.44136831164089,1.43598613500131,
-7.76450570621253));
#366025=CARTESIAN_POINT('Ctrl Pts',(-1.98707527820992,2.01844704832099,
-7.79196266491878));
#366026=CARTESIAN_POINT('Ctrl Pts',(-1.39756088034447,2.46348708795637,
-7.8194137894634));
#366027=CARTESIAN_POINT('Ctrl Pts',(-0.710881081634362,2.74170412714945,
-7.84704636495045));
#366028=CARTESIAN_POINT('Ctrl Pts',(0.0221378788343896,2.83233850612441,
-7.87451146130275));
#366029=CARTESIAN_POINT('Ctrl Pts',(0.753693185451086,2.73018185071023,
-7.90193724347128));
#366030=CARTESIAN_POINT('Ctrl Pts',(1.43623604645724,2.44132953435746,-7.92960016599444));
#366031=CARTESIAN_POINT('Ctrl Pts',(1.96972754709332,2.02444453015913,-7.95479275010049));
#366032=CARTESIAN_POINT('Ctrl Pts',(2.35530318309127,1.54946734602988,-7.97759034640265));
#366033=CARTESIAN_POINT('Ctrl Pts',(2.61262613808022,1.05037578999858,-7.9984674292579));
#366034=CARTESIAN_POINT('Ctrl Pts',(2.76839001336968,0.552800283700582,
-8.01843767560678));
#366035=CARTESIAN_POINT('Ctrl Pts',(2.80021499480674,0.108538122595088,
-8.03388883389828));
#366036=CARTESIAN_POINT('Ctrl Pts',(2.80021499480674,-0.0219216792995908,
-8.0396015159865));
#366037=CARTESIAN_POINT('Ctrl Pts',(2.7998363224979,0.0349606549171637,
-8.01981010684661));
#366038=CARTESIAN_POINT('Ctrl Pts',(2.7998363224979,-0.108453789702572,
-8.02609005758295));
#366039=CARTESIAN_POINT('Ctrl Pts',(2.76770770092932,-0.554475300665122,
-8.04161041709402));
#366040=CARTESIAN_POINT('Ctrl Pts',(2.61230104920345,-1.04994348735895,
-8.06150470700589));
#366041=CARTESIAN_POINT('Ctrl Pts',(2.35499212095577,-1.5493099165356,-8.08239384111292));
#366042=CARTESIAN_POINT('Ctrl Pts',(1.96948131702204,-2.02412699417522,
-8.10518795929102));
#366043=CARTESIAN_POINT('Ctrl Pts',(1.43606137034988,-2.44099583455896,
-8.1303818337545));
#366044=CARTESIAN_POINT('Ctrl Pts',(0.753613249673498,-2.7298044063241,
-8.15804434422187));
#366045=CARTESIAN_POINT('Ctrl Pts',(0.0221607848766011,-2.83195604538419,
-8.18547015377513));
#366046=CARTESIAN_POINT('Ctrl Pts',(-0.710763089306898,-2.74133925166452,
-8.21293536328677));
#366047=CARTESIAN_POINT('Ctrl Pts',(-1.39735180486206,-2.46316525092768,
-8.24056787474674));
#366048=CARTESIAN_POINT('Ctrl Pts',(-1.9867882252217,-2.01819243450698,
-8.26801892009786));
#366049=CARTESIAN_POINT('Ctrl Pts',(-2.44102701245388,-1.43581160139486,
-8.2954760307671));
#366050=CARTESIAN_POINT('Ctrl Pts',(-2.72979268536681,-0.753649988228477,
-8.32310562488017));
#366051=CARTESIAN_POINT('Ctrl Pts',(-2.83194900848818,-0.022207241173352,
-8.35056035976573));
#366052=CARTESIAN_POINT('Ctrl Pts',(-2.74133888936392,0.710795480178799,
-8.37801577635552));
#366053=CARTESIAN_POINT('Ctrl Pts',(-2.4631658691281,1.3973450383548,-8.4056453623318));
#366054=CARTESIAN_POINT('Ctrl Pts',(-2.0181913618354,1.98678420052489,-8.43310180787527));
#366055=CARTESIAN_POINT('Ctrl Pts',(-1.43582178716812,2.44103031792683,
-8.4605535408052));
#366056=CARTESIAN_POINT('Ctrl Pts',(-0.753616702679641,2.7297964193171,
-8.48818595954062));
#366057=CARTESIAN_POINT('Ctrl Pts',(-0.0222544062348159,2.83192570994805,
-8.51565069030184));
#366058=CARTESIAN_POINT('Ctrl Pts',(0.710769507993571,2.74139122758401,
-8.54307702242869));
#366059=CARTESIAN_POINT('Ctrl Pts',(1.39758336815266,2.4631211079265,-8.5707395161615));
#366060=CARTESIAN_POINT('Ctrl Pts',(1.93746427579644,2.05471988808546,-8.59593214237152));
#366061=CARTESIAN_POINT('Ctrl Pts',(2.33041781164643,1.58599477455527,-8.61873057100975));
#366062=CARTESIAN_POINT('Ctrl Pts',(2.59583452983605,1.0910815303924,-8.63960593440206));
#366063=CARTESIAN_POINT('Ctrl Pts',(2.75797391874601,0.595981365328419,
-8.65957756239152));
#366064=CARTESIAN_POINT('Ctrl Pts',(2.79978489023148,0.152404921343189,
-8.67502839375386));
#366065=CARTESIAN_POINT('Ctrl Pts',(2.79978489023148,0.0219451194485099,
-8.68074107584208));
#366066=CARTESIAN_POINT('Ctrl Pts',(1.99983638908381,0.0349322317807904,
-8.0195498399348));
#366067=CARTESIAN_POINT('Ctrl Pts',(1.99983638908381,-0.10202602676277,
-8.02554708183654));
#366068=CARTESIAN_POINT('Ctrl Pts',(1.97826023278427,-0.374998458759011,
-8.04149750289518));
#366069=CARTESIAN_POINT('Ctrl Pts',(1.86797590755627,-0.748764460301907,
-8.06112897846829));
#366070=CARTESIAN_POINT('Ctrl Pts',(1.68561151450438,-1.10015061289253,
-8.08203775324541));
#366071=CARTESIAN_POINT('Ctrl Pts',(1.41165495945895,-1.44156834906321,
-8.10493617015518));
#366072=CARTESIAN_POINT('Ctrl Pts',(1.03047577828238,-1.74058787531436,
-8.13018098020224));
#366073=CARTESIAN_POINT('Ctrl Pts',(0.544916715445223,-1.94793268220013,
-8.15762809500727));
#366074=CARTESIAN_POINT('Ctrl Pts',(0.0221827178159963,-2.02289026809774,
-8.18519084627103));
#366075=CARTESIAN_POINT('Ctrl Pts',(-0.502090027370269,-1.95945608733342,
-8.21271232019691));
#366076=CARTESIAN_POINT('Ctrl Pts',(-0.992083838417867,-1.76270006106949,
-8.24018259789098));
#366077=CARTESIAN_POINT('Ctrl Pts',(-1.4147054776909,-1.44608180030657,
-8.26772003513789));
#366078=CARTESIAN_POINT('Ctrl Pts',(-1.74058220612872,-1.03051305966975,
-8.29525381080208));
#366079=CARTESIAN_POINT('Ctrl Pts',(-1.94792527911454,-0.54490922807225,
-8.32272397147271));
#366080=CARTESIAN_POINT('Ctrl Pts',(-2.02288104093964,-0.0221860622005593,
-8.3502586988329));
#366081=CARTESIAN_POINT('Ctrl Pts',(-1.95946064553349,0.502094730808056,
-8.37779410728247));
#366082=CARTESIAN_POINT('Ctrl Pts',(-1.76270043378214,0.992082445780963,
-8.40526426032094));
#366083=CARTESIAN_POINT('Ctrl Pts',(-1.4460786623108,1.41470354935293,-8.43279736946537));
#366084=CARTESIAN_POINT('Ctrl Pts',(-1.03051788283039,1.74058563617661,
-8.46033550064529));
#366085=CARTESIAN_POINT('Ctrl Pts',(-0.544903604360224,1.94792449639017,
-8.48780566031878));
#366086=CARTESIAN_POINT('Ctrl Pts',(-0.0221901307924648,2.02285846845712,
-8.51532675052651));
#366087=CARTESIAN_POINT('Ctrl Pts',(0.502112905323441,1.95951419733875,
-8.5428896703966));
#366088=CARTESIAN_POINT('Ctrl Pts',(0.992033718187761,1.76267182698944,
-8.57033808767502));
#366089=CARTESIAN_POINT('Ctrl Pts',(1.37966890086895,1.47220110119364,-8.59557713282226));
#366090=CARTESIAN_POINT('Ctrl Pts',(1.66105846219667,1.13661442398405,-8.61849276017575));
#366091=CARTESIAN_POINT('Ctrl Pts',(1.85153124055178,0.790568741290481,
-8.63934277351964));
#366092=CARTESIAN_POINT('Ctrl Pts',(1.96844225278085,0.414017589463527,
-8.65921974028535));
#366093=CARTESIAN_POINT('Ctrl Pts',(1.99978500519319,0.152400794214044,
-8.67468495623063));
#366094=CARTESIAN_POINT('Ctrl Pts',(1.99978500519318,0.0219216792995357,
-8.68039848401339));
#366095=CARTESIAN_POINT('Ctrl Pts',(1.19983645566973,0.0349038086444169,
-8.01928957302298));
#366096=CARTESIAN_POINT('Ctrl Pts',(1.19983645566973,-0.0955982638229683,
-8.02500410609012));
#366097=CARTESIAN_POINT('Ctrl Pts',(1.18881276463922,-0.1955216168529,-8.04138458869635));
#366098=CARTESIAN_POINT('Ctrl Pts',(1.12365076590908,-0.447585433244864,
-8.06075324993069));
#366099=CARTESIAN_POINT('Ctrl Pts',(1.016230908053,-0.650991309249464,-8.0816816653779));
#366100=CARTESIAN_POINT('Ctrl Pts',(0.853828601895857,-0.859009703951189,
-8.10468438101933));
#366101=CARTESIAN_POINT('Ctrl Pts',(0.624890186214873,-1.04017991606976,
-8.12998012664998));
#366102=CARTESIAN_POINT('Ctrl Pts',(0.336220181216949,-1.16606095807615,
-8.15721184579269));
#366103=CARTESIAN_POINT('Ctrl Pts',(0.0222046507553913,-1.21382449081129,
-8.18491153876691));
#366104=CARTESIAN_POINT('Ctrl Pts',(-0.29341696543364,-1.17757292300231,
-8.21248927710705));
#366105=CARTESIAN_POINT('Ctrl Pts',(-0.586815871973671,-1.0622348712113,
-8.23979732103521));
#366106=CARTESIAN_POINT('Ctrl Pts',(-0.842622730160096,-0.873971166106157,
-8.26742115017792));
#366107=CARTESIAN_POINT('Ctrl Pts',(-1.04013739980356,-0.625214517944632,
-8.29503159083705));
#366108=CARTESIAN_POINT('Ctrl Pts',(-1.16605787286226,-0.336168467916023,
-8.32234231806526));
#366109=CARTESIAN_POINT('Ctrl Pts',(-1.2138130733911,-0.0221648832277664,
-8.34995703790007));
#366110=CARTESIAN_POINT('Ctrl Pts',(-1.17758240170305,0.293393981437313,
-8.37757243820942));
#366111=CARTESIAN_POINT('Ctrl Pts',(-1.06223499843619,0.586819853207128,
-8.40488315831008));
#366112=CARTESIAN_POINT('Ctrl Pts',(-0.873965962786202,0.842622898180978,
-8.43249293105548));
#366113=CARTESIAN_POINT('Ctrl Pts',(-0.625213978492663,1.04014095442639,
-8.46011746048537));
#366114=CARTESIAN_POINT('Ctrl Pts',(-0.336190506040807,1.16605257346324,
-8.48742536109694));
#366115=CARTESIAN_POINT('Ctrl Pts',(-0.0221258553501136,1.21379122696619,
-8.51500281075118));
#366116=CARTESIAN_POINT('Ctrl Pts',(0.293456302653311,1.17763716709349,
-8.54270231836451));
#366117=CARTESIAN_POINT('Ctrl Pts',(0.586484068222858,1.06222254605237,
-8.56993665918854));
#366118=CARTESIAN_POINT('Ctrl Pts',(0.821873525941461,0.889682314301827,
-8.59522212327301));
#366119=CARTESIAN_POINT('Ctrl Pts',(0.991699112746911,0.687234073412837,
-8.61825494934175));
#366120=CARTESIAN_POINT('Ctrl Pts',(1.1072279512675,0.490055952188566,-8.63907961263722));
#366121=CARTESIAN_POINT('Ctrl Pts',(1.17891058681569,0.232053813598634,
-8.65886191817918));
#366122=CARTESIAN_POINT('Ctrl Pts',(1.19978512015489,0.152396667084899,
-8.6743415187074));
#366123=CARTESIAN_POINT('Ctrl Pts',(1.19978512015489,0.0218982391505614,
-8.6800558921847));
#366124=CARTESIAN_POINT('Ctrl Pts',(1.20016374408796,-0.0349890780535269,
-7.37928962624154));
#366125=CARTESIAN_POINT('Ctrl Pts',(1.20016374408796,-0.152578778368561,
-7.38443874163948));
#366126=CARTESIAN_POINT('Ctrl Pts',(1.17911220611093,-0.232722898983027,
-7.39997547020929));
#366127=CARTESIAN_POINT('Ctrl Pts',(1.1075697276325,-0.490223236218595,
-7.41968691295851));
#366128=CARTESIAN_POINT('Ctrl Pts',(0.99197768152021,-0.687507626341548,
-7.44052238955959));
#366129=CARTESIAN_POINT('Ctrl Pts',(0.822094024457586,-0.889997593033309,
-7.46355198851942));
#366130=CARTESIAN_POINT('Ctrl Pts',(0.586621297546092,-1.06258644476029,
-7.48883857285657));
#366131=CARTESIAN_POINT('Ctrl Pts',(0.293494109151169,-1.17802345829468,
-7.51607274052479));
#366132=CARTESIAN_POINT('Ctrl Pts',(-0.022187686898918,-1.21417424150576,
-7.54377213707865));
#366133=CARTESIAN_POINT('Ctrl Pts',(-0.336350160913456,-1.16640636249992,
-7.5713496486398));
#366134=CARTESIAN_POINT('Ctrl Pts',(-0.625460469375504,-1.04044098900401,
-7.59865763798262));
#366135=CARTESIAN_POINT('Ctrl Pts',(-0.874280464948115,-0.842850034402287,
-7.62628200750612));
#366136=CARTESIAN_POINT('Ctrl Pts',(-1.06259809494344,-0.586957088863615,
-7.65389185873512));
#366137=CARTESIAN_POINT('Ctrl Pts',(-1.17796883239637,-0.293431870475487,
-7.68120265465688));
#366138=CARTESIAN_POINT('Ctrl Pts',(-1.21419607859374,0.0222266596598858,
-7.70881790257747));
#366139=CARTESIAN_POINT('Ctrl Pts',(-1.16641165708731,0.33632818669979,
-7.73643269887416));
#366140=CARTESIAN_POINT('Ctrl Pts',(-1.04043744094898,0.625460949710965,
-7.76374350219705));
#366141=CARTESIAN_POINT('Ctrl Pts',(-0.842849879160721,0.874285746196179,
-7.7913537880894));
#366142=CARTESIAN_POINT('Ctrl Pts',(-0.58695307166902,1.06259772372267,
-7.81897770917568));
#366143=CARTESIAN_POINT('Ctrl Pts',(-0.293454884995528,1.17796028400778,
-7.846285766388));
#366144=CARTESIAN_POINT('Ctrl Pts',(0.0222664297190919,1.21420401301477,
-7.87386358219558));
#366145=CARTESIAN_POINT('Ctrl Pts',(0.336379980110826,1.16642782799535,
-7.90156253775294));
#366146=CARTESIAN_POINT('Ctrl Pts',(0.625136746527436,1.04043083158176,
-7.9287973151914));
#366147=CARTESIAN_POINT('Ctrl Pts',(0.854136797238339,0.859407427363523,
-7.95408271037797));
#366148=CARTESIAN_POINT('Ctrl Pts',(1.01658448419176,0.650705368151239,
-7.97711478064143));
#366149=CARTESIAN_POINT('Ctrl Pts',(1.12401955951167,0.449355030494726,
-7.99794089648783));
#366150=CARTESIAN_POINT('Ctrl Pts',(1.18932668143936,0.188854714016773,
-8.01772282037956));
#366151=CARTESIAN_POINT('Ctrl Pts',(1.20021522473016,0.108568494376457,
-8.03320026746274));
#366152=CARTESIAN_POINT('Ctrl Pts',(1.20021522473015,-0.0219685595975393,
-8.03891633232913));
#366153=CARTESIAN_POINT('Ctrl Pts',(2.00016367750204,-0.0349606549171534,
-7.37954989315335));
#366154=CARTESIAN_POINT('Ctrl Pts',(2.00016367750204,-0.165462727384539,
-7.38526442622049));
#366155=CARTESIAN_POINT('Ctrl Pts',(1.96855967425598,-0.409173319918984,
-7.39995586097472));
#366156=CARTESIAN_POINT('Ctrl Pts',(1.85189486927969,-0.792213245836797,
-7.42009815347362));
#366157=CARTESIAN_POINT('Ctrl Pts',(1.6613582879716,-1.13645205609876,-7.44086906835104));
#366158=CARTESIAN_POINT('Ctrl Pts',(1.37992038202068,-1.47263550497672,
-7.46380724865708));
#366159=CARTESIAN_POINT('Ctrl Pts',(0.992206889613594,-1.76297069041634,
-7.48903838801854));
#366160=CARTESIAN_POINT('Ctrl Pts',(0.502190643379444,-1.95990154002328,
-7.51648926813145));
#366161=CARTESIAN_POINT('Ctrl Pts',(-0.0222096198383131,-2.0232383143754,
-7.54405136994835));
#366162=CARTESIAN_POINT('Ctrl Pts',(-0.545023222850085,-1.94828998299833,
-7.57157271170469));
#366163=CARTESIAN_POINT('Ctrl Pts',(-1.0307284358197,-1.74090605654878,
-7.59904290948243));
#366164=CARTESIAN_POINT('Ctrl Pts',(-1.44636321247892,-1.41496070139146,
-7.62658089390187));
#366165=CARTESIAN_POINT('Ctrl Pts',(-1.7630429012686,-0.992255621812916,
-7.65411407831587));
#366166=CARTESIAN_POINT('Ctrl Pts',(-1.95983623864864,-0.502172632985278,
-7.68158430816739));
#366167=CARTESIAN_POINT('Ctrl Pts',(-2.02326404614228,0.0222054813197516,
-7.70911956348259));
#366168=CARTESIAN_POINT('Ctrl Pts',(-1.94828990091774,0.545028935894718,
-7.73665436795491));
#366169=CARTESIAN_POINT('Ctrl Pts',(-1.74090287629493,1.03072354235614,
-7.76412460420479));
#366170=CARTESIAN_POINT('Ctrl Pts',(-1.41496257868532,1.44636639725859,
-7.79165822650409));
#366171=CARTESIAN_POINT('Ctrl Pts',(-0.992256976006747,1.76304240583952,
-7.81919574931953));
#366172=CARTESIAN_POINT('Ctrl Pts',(-0.502167983314945,1.95983220557862,
-7.84666606566923));
#366173=CARTESIAN_POINT('Ctrl Pts',(0.0222021542767409,2.02327125956959,
-7.87418752174917));
#366174=CARTESIAN_POINT('Ctrl Pts',(0.545036582780956,1.94830483935279,
-7.90174989061211));
#366175=CARTESIAN_POINT('Ctrl Pts',(1.03068639649234,1.74088018296961,-7.92919874059292));
#366176=CARTESIAN_POINT('Ctrl Pts',(1.41193217216583,1.44192597876132,-7.95443773023923));
#366177=CARTESIAN_POINT('Ctrl Pts',(1.68594383364152,1.10008635709056,-7.97735256352204));
#366178=CARTESIAN_POINT('Ctrl Pts',(1.86832284879594,0.749865410246654,
-7.99820416287286));
#366179=CARTESIAN_POINT('Ctrl Pts',(1.97885834740452,0.370827498858678,
-8.01808024799317));
#366180=CARTESIAN_POINT('Ctrl Pts',(2.00021510976845,0.108553308485772,
-8.03354455068052));
#366181=CARTESIAN_POINT('Ctrl Pts',(2.00021510976845,-0.0219451194485651,
-8.03925892415782));
#459204=UNCERTAINTY_MEASURE_WITH_UNIT(LENGTH_MEASURE(0.01),#459243,
'DISTANCE_ACCURACY_VALUE',
'Maximum model space distance between geometric entities at asserted c
onnectivities');
#459216=UNCERTAINTY_MEASURE_WITH_UNIT(LENGTH_MEASURE(0.01),#459243,
'DISTANCE_ACCURACY_VALUE',
'Maximum model space distance between geometric entities at asserted c
onnectivities');
#459230=(
GEOMETRIC_REPRESENTATION_CONTEXT(3)
GLOBAL_UNCERTAINTY_ASSIGNED_CONTEXT((#459204))
GLOBAL_UNIT_ASSIGNED_CONTEXT((#459243,#459245,#459246))
REPRESENTATION_CONTEXT('','3D')
);
#459242=(
GEOMETRIC_REPRESENTATION_CONTEXT(3)
GLOBAL_UNCERTAINTY_ASSIGNED_CONTEXT((#459216))
GLOBAL_UNIT_ASSIGNED_CONTEXT((#459243,#459245,#459246))
REPRESENTATION_CONTEXT('','3D')
);
#459243=(
LENGTH_UNIT()
NAMED_UNIT(*)
SI_UNIT(.MILLI.,.METRE.)
);
#459245=(
NAMED_UNIT(*)
PLANE_ANGLE_UNIT()
SI_UNIT($,.RADIAN.)
);
#459246=(
NAMED_UNIT(*)
SI_UNIT($,.STERADIAN.)
SOLID_ANGLE_UNIT()
);
#459260=SHAPE_DEFINITION_REPRESENTATION(#459285,#459341);
#459285=PRODUCT_DEFINITION_SHAPE('',$,#459367);
#459341=SHAPE_REPRESENTATION('',(#99154),#459230);
#459353=PRODUCT_DEFINITION_CONTEXT('part definition',#459430,'design');
#459367=PRODUCT_DEFINITION('Compression Spring 0.8x5x10',
'Compression Spring 0.8x5x10',#459392,#459353);
#459392=PRODUCT_DEFINITION_FORMATION('',$,#459445);
#459430=APPLICATION_CONTEXT(
'Core Data for Automotive Mechanical Design Process');
#459431=PRODUCT_CONTEXT('part definition',#459430,'mechanical');
#459445=PRODUCT('Compression Spring 0.8x5x10',
'Compression Spring 0.8x5x10',$,(#459431));
#459520=COLOUR_RGB('Grey',0.48,0.52,0.57);
#459521=FILL_AREA_STYLE_COLOUR('',#459520);
#459522=FILL_AREA_STYLE('',(#459521));
#459523=SURFACE_STYLE_FILL_AREA(#459522);
#459524=SURFACE_SIDE_STYLE('',(#459523));
#459525=SURFACE_STYLE_USAGE(.BOTH.,#459524);
#459526=PRESENTATION_STYLE_ASSIGNMENT((#459525));
ENDSEC;
END-ISO-10303-21;
